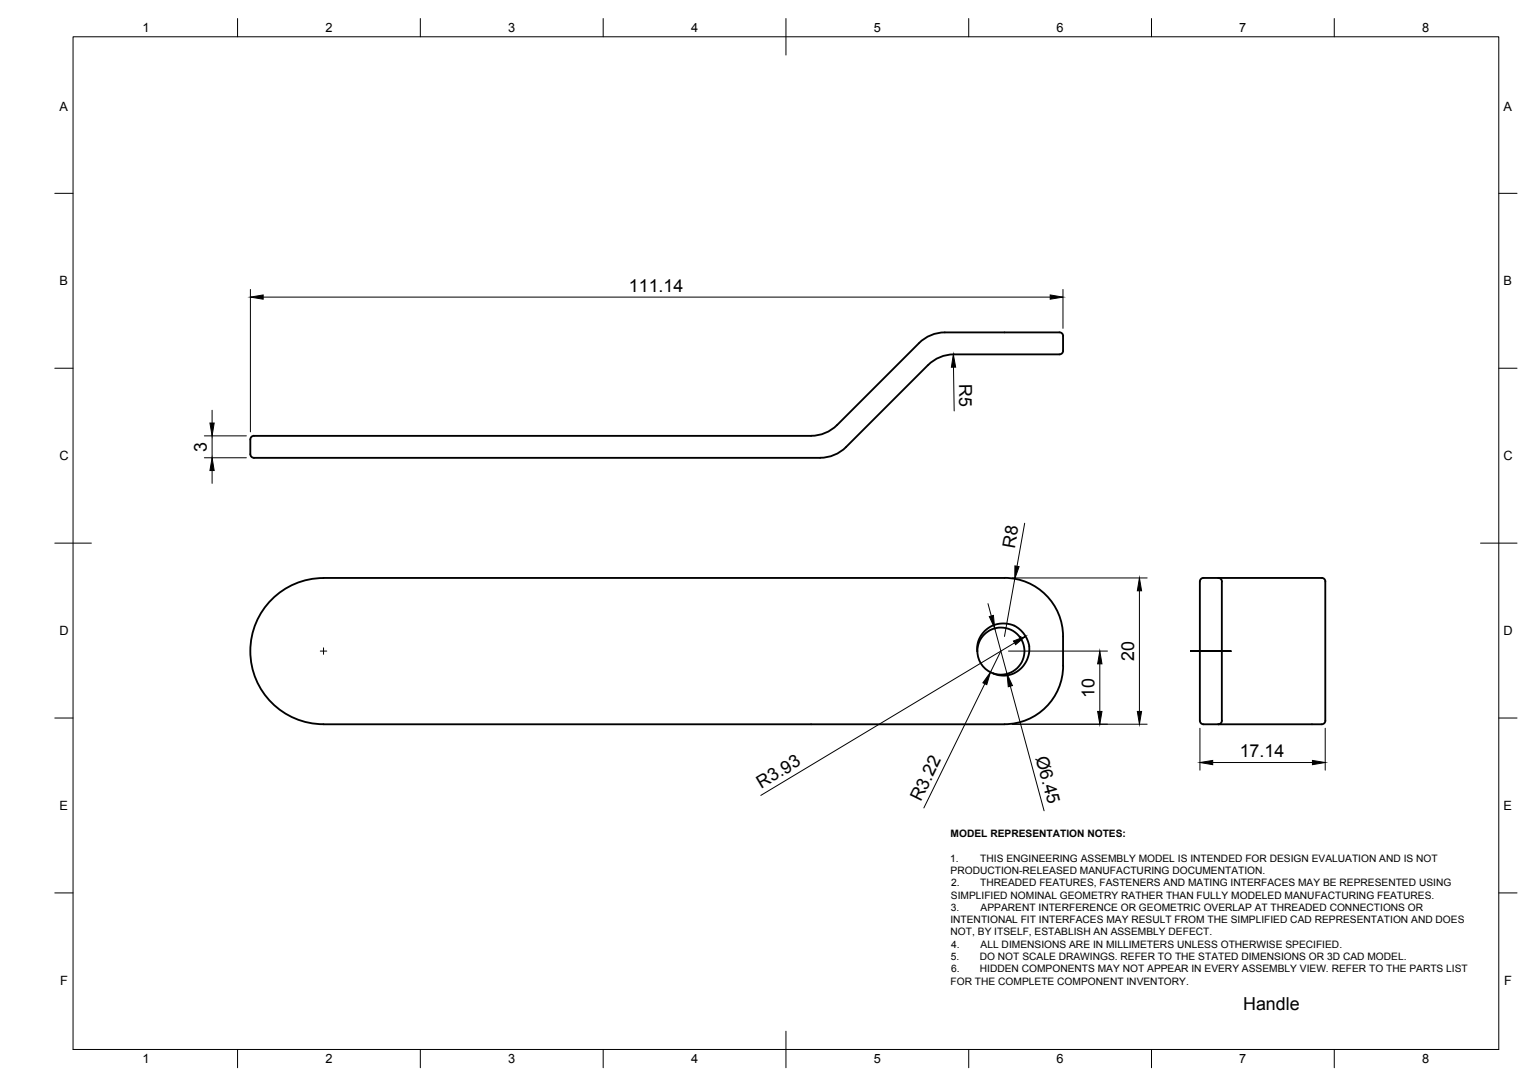
ISO-10303-21;
HEADER;
/* Generated by software containing ST-Developer
 * from STEP Tools, Inc. (www.steptools.com) 
 */

FILE_DESCRIPTION(
/* description */ (''),
/* implementation_level */ '2;1');

FILE_NAME(
/* name */ 'Handle.step',
/* time_stamp */ '2026-10-06T12:47:13-07:00',
/* author */ (''),
/* organization */ (''),
/* preprocessor_version */ 'ST-DEVELOPER v20.2',
/* originating_system */ 'Autodesk Translation Framework v15.15.0.0',
/* authorisation */ '');

FILE_SCHEMA (('AUTOMOTIVE_DESIGN { 1 0 10303 214 3 1 1 }'));
ENDSEC;

DATA;
#10=MECHANICAL_DESIGN_GEOMETRIC_PRESENTATION_REPRESENTATION('',(#74),#42667);
#56=SHAPE_REPRESENTATION_RELATIONSHIP('SRR','None',#42709,#65);
#65=ADVANCED_BREP_SHAPE_REPRESENTATION('',(#83),#42665);
#74=STYLED_ITEM('',(#42756),#83);
#83=MANIFOLD_SOLID_BREP('Body1',#4039);
#90=B_SPLINE_SURFACE_WITH_KNOTS('',3,3,((#34754,#34755,#34756,#34757,#34758,
#34759,#34760,#34761,#34762,#34763,#34764,#34765,#34766,#34767,#34768,#34769,
#34770,#34771,#34772,#34773,#34774,#34775,#34776,#34777,#34778,#34779,#34780,
#34781,#34782,#34783,#34784,#34785,#34786,#34787,#34788,#34789,#34790,#34791,
#34792,#34793,#34794,#34795,#34796,#34797,#34798,#34799,#34800,#34801,#34802,
#34803,#34804,#34805,#34806,#34807,#34808,#34809,#34810,#34811,#34812,#34813,
#34814,#34815,#34816,#34817,#34818,#34819,#34820,#34821,#34822,#34823,#34824,
#34825,#34826,#34827,#34828,#34829,#34830,#34831,#34832,#34833,#34834,#34835,
#34836,#34837,#34838,#34839,#34840,#34841,#34842,#34843,#34844,#34845,#34846,
#34847,#34848,#34849,#34850,#34851,#34852,#34853,#34854,#34855,#34856,#34857,
#34858,#34859,#34860,#34861,#34862,#34863,#34864,#34865,#34866,#34867,#34868,
#34869,#34870,#34871,#34872,#34873,#34874,#34875,#34876,#34877,#34878,#34879,
#34880,#34881,#34882,#34883,#34884,#34885,#34886,#34887,#34888,#34889,#34890,
#34891,#34892,#34893,#34894,#34895,#34896,#34897,#34898,#34899,#34900,#34901,
#34902,#34903,#34904,#34905,#34906,#34907,#34908,#34909,#34910,#34911,#34912,
#34913,#34914,#34915,#34916,#34917,#34918,#34919,#34920,#34921,#34922,#34923,
#34924,#34925,#34926,#34927,#34928,#34929,#34930,#34931,#34932,#34933,#34934),
(#34935,#34936,#34937,#34938,#34939,#34940,#34941,#34942,#34943,#34944,
#34945,#34946,#34947,#34948,#34949,#34950,#34951,#34952,#34953,#34954,#34955,
#34956,#34957,#34958,#34959,#34960,#34961,#34962,#34963,#34964,#34965,#34966,
#34967,#34968,#34969,#34970,#34971,#34972,#34973,#34974,#34975,#34976,#34977,
#34978,#34979,#34980,#34981,#34982,#34983,#34984,#34985,#34986,#34987,#34988,
#34989,#34990,#34991,#34992,#34993,#34994,#34995,#34996,#34997,#34998,#34999,
#35000,#35001,#35002,#35003,#35004,#35005,#35006,#35007,#35008,#35009,#35010,
#35011,#35012,#35013,#35014,#35015,#35016,#35017,#35018,#35019,#35020,#35021,
#35022,#35023,#35024,#35025,#35026,#35027,#35028,#35029,#35030,#35031,#35032,
#35033,#35034,#35035,#35036,#35037,#35038,#35039,#35040,#35041,#35042,#35043,
#35044,#35045,#35046,#35047,#35048,#35049,#35050,#35051,#35052,#35053,#35054,
#35055,#35056,#35057,#35058,#35059,#35060,#35061,#35062,#35063,#35064,#35065,
#35066,#35067,#35068,#35069,#35070,#35071,#35072,#35073,#35074,#35075,#35076,
#35077,#35078,#35079,#35080,#35081,#35082,#35083,#35084,#35085,#35086,#35087,
#35088,#35089,#35090,#35091,#35092,#35093,#35094,#35095,#35096,#35097,#35098,
#35099,#35100,#35101,#35102,#35103,#35104,#35105,#35106,#35107,#35108,#35109,
#35110,#35111,#35112,#35113,#35114,#35115),(#35116,#35117,#35118,#35119,
#35120,#35121,#35122,#35123,#35124,#35125,#35126,#35127,#35128,#35129,#35130,
#35131,#35132,#35133,#35134,#35135,#35136,#35137,#35138,#35139,#35140,#35141,
#35142,#35143,#35144,#35145,#35146,#35147,#35148,#35149,#35150,#35151,#35152,
#35153,#35154,#35155,#35156,#35157,#35158,#35159,#35160,#35161,#35162,#35163,
#35164,#35165,#35166,#35167,#35168,#35169,#35170,#35171,#35172,#35173,#35174,
#35175,#35176,#35177,#35178,#35179,#35180,#35181,#35182,#35183,#35184,#35185,
#35186,#35187,#35188,#35189,#35190,#35191,#35192,#35193,#35194,#35195,#35196,
#35197,#35198,#35199,#35200,#35201,#35202,#35203,#35204,#35205,#35206,#35207,
#35208,#35209,#35210,#35211,#35212,#35213,#35214,#35215,#35216,#35217,#35218,
#35219,#35220,#35221,#35222,#35223,#35224,#35225,#35226,#35227,#35228,#35229,
#35230,#35231,#35232,#35233,#35234,#35235,#35236,#35237,#35238,#35239,#35240,
#35241,#35242,#35243,#35244,#35245,#35246,#35247,#35248,#35249,#35250,#35251,
#35252,#35253,#35254,#35255,#35256,#35257,#35258,#35259,#35260,#35261,#35262,
#35263,#35264,#35265,#35266,#35267,#35268,#35269,#35270,#35271,#35272,#35273,
#35274,#35275,#35276,#35277,#35278,#35279,#35280,#35281,#35282,#35283,#35284,
#35285,#35286,#35287,#35288,#35289,#35290,#35291,#35292,#35293,#35294,#35295,
#35296),(#35297,#35298,#35299,#35300,#35301,#35302,#35303,#35304,#35305,
#35306,#35307,#35308,#35309,#35310,#35311,#35312,#35313,#35314,#35315,#35316,
#35317,#35318,#35319,#35320,#35321,#35322,#35323,#35324,#35325,#35326,#35327,
#35328,#35329,#35330,#35331,#35332,#35333,#35334,#35335,#35336,#35337,#35338,
#35339,#35340,#35341,#35342,#35343,#35344,#35345,#35346,#35347,#35348,#35349,
#35350,#35351,#35352,#35353,#35354,#35355,#35356,#35357,#35358,#35359,#35360,
#35361,#35362,#35363,#35364,#35365,#35366,#35367,#35368,#35369,#35370,#35371,
#35372,#35373,#35374,#35375,#35376,#35377,#35378,#35379,#35380,#35381,#35382,
#35383,#35384,#35385,#35386,#35387,#35388,#35389,#35390,#35391,#35392,#35393,
#35394,#35395,#35396,#35397,#35398,#35399,#35400,#35401,#35402,#35403,#35404,
#35405,#35406,#35407,#35408,#35409,#35410,#35411,#35412,#35413,#35414,#35415,
#35416,#35417,#35418,#35419,#35420,#35421,#35422,#35423,#35424,#35425,#35426,
#35427,#35428,#35429,#35430,#35431,#35432,#35433,#35434,#35435,#35436,#35437,
#35438,#35439,#35440,#35441,#35442,#35443,#35444,#35445,#35446,#35447,#35448,
#35449,#35450,#35451,#35452,#35453,#35454,#35455,#35456,#35457,#35458,#35459,
#35460,#35461,#35462,#35463,#35464,#35465,#35466,#35467,#35468,#35469,#35470,
#35471,#35472,#35473,#35474,#35475,#35476,#35477)),.UNSPECIFIED.,.F.,.F.,
 .F.,(4,4),(4,1,1,1,1,1,1,1,1,1,1,1,1,1,1,1,1,1,1,1,1,1,1,1,1,1,1,1,1,1,
1,1,1,1,1,1,1,1,1,1,1,1,1,1,1,1,1,1,1,1,1,1,1,1,1,1,1,1,1,1,1,1,1,1,1,1,
1,1,1,1,1,1,1,1,1,1,1,1,1,1,1,1,1,1,1,1,1,1,1,1,1,1,1,1,1,1,1,1,1,1,1,1,
1,1,1,1,1,1,1,1,1,1,1,1,1,1,1,1,1,1,1,1,1,1,1,1,1,1,1,1,1,1,1,1,1,1,1,1,
1,1,1,1,1,1,1,1,1,1,1,1,1,1,1,1,1,1,1,1,1,1,1,1,1,1,1,1,1,1,1,1,1,1,1,1,
1,1,1,1,4),(-0.000650925100349628,0.0823958707828885),(8.31473274985812,
9.3146787622095,10.3146247745609,11.3145707869122,12.3145167992636,13.314462811615,
14.3144088239664,15.3143548363177,16.3143008486691,17.3142468610205,18.3141928733718,
19.3141388857232,20.3140848980746,21.314030910426,22.3139769227773,23.3139229351287,
24.3138689474801,25.3138149598315,26.3137609721828,27.3137069845342,28.3136529968856,
29.3135990092369,30.3135450215883,31.3134910339397,32.3134370462911,33.3133830586424,
34.3133290709938,35.3132750833452,36.3132210956965,37.3131671080479,38.3131131203993,
39.3130591327507,40.313005145102,41.3129511574534,42.3128971698048,43.3128431821562,
44.3127891945075,45.3127352068589,46.3126812192103,47.3126272315616,48.312573243913,
49.3125192562644,50.3124652686158,51.3124112809671,52.3123572933185,53.3123033056699,
54.3122493180213,55.3121953303726,56.312141342724,57.3120873550754,58.3120333674267,
59.3119793797781,60.3119253921295,61.3118714044809,62.3118174168322,63.3117634291836,
64.311709441535,65.3116554538863,66.3116014662377,67.3115474785891,68.3114934909405,
69.3114395032918,70.3113855156432,71.3113315279946,72.311277540346,73.3112235526973,
74.3111695650487,75.3111155774001,76.3110615897514,77.3110076021028,78.3109536144542,
79.3108996268056,80.3108456391569,81.3107916515083,82.3107376638597,83.3106836762111,
84.3106296885624,85.3105757009138,86.3105217132652,87.3104677256165,88.3104137379679,
89.3103597503193,90.3103057626707,91.310251775022,92.3101977873734,93.3101437997248,
94.3100898120761,95.3100358244275,96.3099818367789,97.3099278491303,98.3098738614816,
99.309819873833,100.309765886184,101.309711898536,102.309657910887,103.309603923238,
104.30954993559,105.309495947941,106.309441960293,107.309387972644,108.309333984995,
109.309279997347,110.309226009698,111.309172022049,112.309118034401,113.309064046752,
114.309010059104,115.308956071455,116.308902083806,117.308848096158,118.308794108509,
119.30874012086,120.308686133212,121.308632145563,122.308578157915,123.308524170266,
124.308470182617,125.308416194969,126.30836220732,127.308308219671,128.308254232023,
129.308200244374,130.308146256726,131.308092269077,132.308038281428,133.30798429378,
134.307930306131,135.307876318482,136.307822330834,137.307768343185,138.307714355537,
139.307660367888,140.307606380239,141.307552392591,142.307498404942,143.307444417293,
144.307390429645,145.307336441996,146.307282454348,147.307228466699,148.30717447905,
149.307120491402,150.307066503753,151.307012516104,152.306958528456,153.306904540807,
154.306850553158,155.30679656551,156.306742577861,157.306688590213,158.306634602564,
159.306580614915,160.306526627267,161.306472639618,162.306418651969,163.306364664321,
164.306310676672,165.306256689024,166.306202701375,167.306148713726,168.306094726078,
169.306040738429,170.30598675078,171.305932763132,172.305878775483,173.305824787835,
174.305770800186,175.305716812537,176.305662824889,177.30560883724,178.305554849591,
179.305500861943,180.305446874294,181.305392886646,182.305338898997,183.305284911348,
184.3052309237,185.305176936051,186.305773873502),.UNSPECIFIED.);
#91=B_SPLINE_SURFACE_WITH_KNOTS('',3,3,((#35967,#35968,#35969,#35970,#35971,
#35972,#35973,#35974,#35975,#35976,#35977,#35978,#35979,#35980,#35981,#35982,
#35983,#35984,#35985,#35986,#35987,#35988,#35989,#35990,#35991,#35992,#35993,
#35994,#35995,#35996,#35997,#35998,#35999,#36000,#36001,#36002,#36003,#36004,
#36005,#36006,#36007,#36008,#36009,#36010,#36011,#36012,#36013,#36014,#36015,
#36016,#36017,#36018,#36019,#36020,#36021,#36022,#36023,#36024,#36025,#36026,
#36027,#36028,#36029,#36030,#36031,#36032,#36033,#36034,#36035,#36036,#36037,
#36038,#36039,#36040,#36041,#36042,#36043,#36044,#36045,#36046,#36047,#36048,
#36049,#36050,#36051,#36052,#36053,#36054,#36055,#36056,#36057,#36058,#36059,
#36060,#36061,#36062,#36063,#36064,#36065,#36066,#36067,#36068,#36069,#36070,
#36071,#36072,#36073,#36074,#36075,#36076,#36077,#36078,#36079,#36080,#36081,
#36082,#36083,#36084,#36085,#36086,#36087,#36088,#36089,#36090,#36091,#36092,
#36093,#36094,#36095,#36096,#36097,#36098,#36099,#36100,#36101,#36102,#36103,
#36104,#36105,#36106,#36107,#36108,#36109,#36110,#36111,#36112,#36113,#36114,
#36115,#36116,#36117,#36118,#36119,#36120,#36121,#36122,#36123,#36124,#36125,
#36126,#36127,#36128,#36129,#36130,#36131,#36132,#36133,#36134,#36135,#36136,
#36137,#36138,#36139,#36140,#36141,#36142,#36143,#36144,#36145,#36146,#36147),
(#36148,#36149,#36150,#36151,#36152,#36153,#36154,#36155,#36156,#36157,
#36158,#36159,#36160,#36161,#36162,#36163,#36164,#36165,#36166,#36167,#36168,
#36169,#36170,#36171,#36172,#36173,#36174,#36175,#36176,#36177,#36178,#36179,
#36180,#36181,#36182,#36183,#36184,#36185,#36186,#36187,#36188,#36189,#36190,
#36191,#36192,#36193,#36194,#36195,#36196,#36197,#36198,#36199,#36200,#36201,
#36202,#36203,#36204,#36205,#36206,#36207,#36208,#36209,#36210,#36211,#36212,
#36213,#36214,#36215,#36216,#36217,#36218,#36219,#36220,#36221,#36222,#36223,
#36224,#36225,#36226,#36227,#36228,#36229,#36230,#36231,#36232,#36233,#36234,
#36235,#36236,#36237,#36238,#36239,#36240,#36241,#36242,#36243,#36244,#36245,
#36246,#36247,#36248,#36249,#36250,#36251,#36252,#36253,#36254,#36255,#36256,
#36257,#36258,#36259,#36260,#36261,#36262,#36263,#36264,#36265,#36266,#36267,
#36268,#36269,#36270,#36271,#36272,#36273,#36274,#36275,#36276,#36277,#36278,
#36279,#36280,#36281,#36282,#36283,#36284,#36285,#36286,#36287,#36288,#36289,
#36290,#36291,#36292,#36293,#36294,#36295,#36296,#36297,#36298,#36299,#36300,
#36301,#36302,#36303,#36304,#36305,#36306,#36307,#36308,#36309,#36310,#36311,
#36312,#36313,#36314,#36315,#36316,#36317,#36318,#36319,#36320,#36321,#36322,
#36323,#36324,#36325,#36326,#36327,#36328),(#36329,#36330,#36331,#36332,
#36333,#36334,#36335,#36336,#36337,#36338,#36339,#36340,#36341,#36342,#36343,
#36344,#36345,#36346,#36347,#36348,#36349,#36350,#36351,#36352,#36353,#36354,
#36355,#36356,#36357,#36358,#36359,#36360,#36361,#36362,#36363,#36364,#36365,
#36366,#36367,#36368,#36369,#36370,#36371,#36372,#36373,#36374,#36375,#36376,
#36377,#36378,#36379,#36380,#36381,#36382,#36383,#36384,#36385,#36386,#36387,
#36388,#36389,#36390,#36391,#36392,#36393,#36394,#36395,#36396,#36397,#36398,
#36399,#36400,#36401,#36402,#36403,#36404,#36405,#36406,#36407,#36408,#36409,
#36410,#36411,#36412,#36413,#36414,#36415,#36416,#36417,#36418,#36419,#36420,
#36421,#36422,#36423,#36424,#36425,#36426,#36427,#36428,#36429,#36430,#36431,
#36432,#36433,#36434,#36435,#36436,#36437,#36438,#36439,#36440,#36441,#36442,
#36443,#36444,#36445,#36446,#36447,#36448,#36449,#36450,#36451,#36452,#36453,
#36454,#36455,#36456,#36457,#36458,#36459,#36460,#36461,#36462,#36463,#36464,
#36465,#36466,#36467,#36468,#36469,#36470,#36471,#36472,#36473,#36474,#36475,
#36476,#36477,#36478,#36479,#36480,#36481,#36482,#36483,#36484,#36485,#36486,
#36487,#36488,#36489,#36490,#36491,#36492,#36493,#36494,#36495,#36496,#36497,
#36498,#36499,#36500,#36501,#36502,#36503,#36504,#36505,#36506,#36507,#36508,
#36509),(#36510,#36511,#36512,#36513,#36514,#36515,#36516,#36517,#36518,
#36519,#36520,#36521,#36522,#36523,#36524,#36525,#36526,#36527,#36528,#36529,
#36530,#36531,#36532,#36533,#36534,#36535,#36536,#36537,#36538,#36539,#36540,
#36541,#36542,#36543,#36544,#36545,#36546,#36547,#36548,#36549,#36550,#36551,
#36552,#36553,#36554,#36555,#36556,#36557,#36558,#36559,#36560,#36561,#36562,
#36563,#36564,#36565,#36566,#36567,#36568,#36569,#36570,#36571,#36572,#36573,
#36574,#36575,#36576,#36577,#36578,#36579,#36580,#36581,#36582,#36583,#36584,
#36585,#36586,#36587,#36588,#36589,#36590,#36591,#36592,#36593,#36594,#36595,
#36596,#36597,#36598,#36599,#36600,#36601,#36602,#36603,#36604,#36605,#36606,
#36607,#36608,#36609,#36610,#36611,#36612,#36613,#36614,#36615,#36616,#36617,
#36618,#36619,#36620,#36621,#36622,#36623,#36624,#36625,#36626,#36627,#36628,
#36629,#36630,#36631,#36632,#36633,#36634,#36635,#36636,#36637,#36638,#36639,
#36640,#36641,#36642,#36643,#36644,#36645,#36646,#36647,#36648,#36649,#36650,
#36651,#36652,#36653,#36654,#36655,#36656,#36657,#36658,#36659,#36660,#36661,
#36662,#36663,#36664,#36665,#36666,#36667,#36668,#36669,#36670,#36671,#36672,
#36673,#36674,#36675,#36676,#36677,#36678,#36679,#36680,#36681,#36682,#36683,
#36684,#36685,#36686,#36687,#36688,#36689,#36690)),.UNSPECIFIED.,.F.,.F.,
 .F.,(4,4),(4,1,1,1,1,1,1,1,1,1,1,1,1,1,1,1,1,1,1,1,1,1,1,1,1,1,1,1,1,1,
1,1,1,1,1,1,1,1,1,1,1,1,1,1,1,1,1,1,1,1,1,1,1,1,1,1,1,1,1,1,1,1,1,1,1,1,
1,1,1,1,1,1,1,1,1,1,1,1,1,1,1,1,1,1,1,1,1,1,1,1,1,1,1,1,1,1,1,1,1,1,1,1,
1,1,1,1,1,1,1,1,1,1,1,1,1,1,1,1,1,1,1,1,1,1,1,1,1,1,1,1,1,1,1,1,1,1,1,1,
1,1,1,1,1,1,1,1,1,1,1,1,1,1,1,1,1,1,1,1,1,1,1,1,1,1,1,1,1,1,1,1,1,1,1,1,
1,1,1,1,4),(-0.00033399260015787,0.082683618112034),(11.6145432153813,12.6151602401062,
13.6151062524576,14.615052264809,15.6149982771603,16.6149442895117,17.6148903018631,
18.6148363142145,19.6147823265658,20.6147283389172,21.6146743512686,22.61462036362,
23.6145663759713,24.6145123883227,25.6144584006741,26.6144044130254,27.6143504253768,
28.6142964377282,29.6142424500796,30.6141884624309,31.6141344747823,32.6140804871337,
33.614026499485,34.6139725118364,35.6139185241878,36.6138645365392,37.6138105488905,
38.6137565612419,39.6137025735933,40.6136485859447,41.613594598296,42.6135406106474,
43.6134866229988,44.6134326353501,45.6133786477015,46.6133246600529,47.6132706724043,
48.6132166847556,49.613162697107,50.6131087094584,51.6130547218097,52.6130007341611,
53.6129467465125,54.6128927588639,55.6128387712152,56.6127847835666,57.612730795918,
58.6126768082694,59.6126228206207,60.6125688329721,61.6125148453235,62.6124608576748,
63.6124068700262,64.6123528823776,65.612298894729,66.6122449070803,67.6121909194317,
68.6121369317831,69.6120829441344,70.6120289564858,71.6119749688372,72.6119209811886,
73.6118669935399,74.6118130058913,75.6117590182427,76.6117050305941,77.6116510429454,
78.6115970552968,79.6115430676482,80.6114890799995,81.6114350923509,82.6113811047023,
83.6113271170537,84.611273129405,85.6112191417564,86.6111651541078,87.6111111664591,
88.6110571788105,89.6110031911619,90.6109492035133,91.6108952158646,92.610841228216,
93.6107872405674,94.6107332529187,95.6106792652701,96.6106252776215,97.6105712899729,
98.6105173023242,99.6104633146756,100.610409327027,101.610355339378,102.61030135173,
103.610247364081,104.610193376432,105.610139388784,106.610085401135,107.610031413487,
108.609977425838,109.609923438189,110.609869450541,111.609815462892,112.609761475243,
113.609707487595,114.609653499946,115.609599512298,116.609545524649,117.609491537,
118.609437549352,119.609383561703,120.609329574054,121.609275586406,122.609221598757,
123.609167611109,124.60911362346,125.609059635811,126.609005648163,127.608951660514,
128.608897672865,129.608843685217,130.608789697568,131.60873570992,132.608681722271,
133.608627734622,134.608573746974,135.608519759325,136.608465771676,137.608411784028,
138.608357796379,139.60830380873,140.608249821082,141.608195833433,142.608141845785,
143.608087858136,144.608033870487,145.607979882839,146.60792589519,147.607871907541,
148.607817919893,149.607763932244,150.607709944596,151.607655956947,152.607601969298,
153.60754798165,154.607493994001,155.607440006352,156.607386018704,157.607332031055,
158.607278043407,159.607224055758,160.607170068109,161.607116080461,162.607062092812,
163.607008105163,164.606954117515,165.606900129866,166.606846142218,167.606792154569,
168.60673816692,169.606684179272,170.606630191623,171.606576203974,172.606522216326,
173.606468228677,174.606414241029,175.60636025338,176.606306265731,177.606252278083,
178.606198290434,179.606144302785,180.606090315137,181.606036327488,182.605982339839,
183.605928352191,184.605874364542,185.605820376894,186.605766389245,187.605712401596,
188.605658413948,189.605604426299),.UNSPECIFIED.);
#304=B_SPLINE_CURVE_WITH_KNOTS('',3,(#33626,#33627,#33628,#33629,#33630,
#33631,#33632,#33633,#33634,#33635,#33636,#33637,#33638,#33639,#33640,#33641,
#33642,#33643,#33644,#33645,#33646,#33647,#33648,#33649,#33650,#33651,#33652,
#33653,#33654,#33655,#33656,#33657,#33658,#33659,#33660,#33661,#33662,#33663,
#33664,#33665,#33666,#33667,#33668,#33669,#33670,#33671,#33672,#33673,#33674,
#33675,#33676,#33677,#33678,#33679,#33680,#33681,#33682,#33683,#33684,#33685,
#33686,#33687,#33688,#33689,#33690,#33691,#33692,#33693,#33694,#33695,#33696,
#33697,#33698,#33699,#33700,#33701,#33702,#33703,#33704,#33705,#33706,#33707,
#33708,#33709,#33710,#33711,#33712,#33713,#33714,#33715,#33716,#33717,#33718,
#33719,#33720,#33721,#33722,#33723,#33724,#33725,#33726,#33727,#33728,#33729,
#33730,#33731),.UNSPECIFIED.,.F.,.F.,(4,3,3,3,3,3,3,3,3,3,3,3,3,3,3,3,3,
3,3,3,3,3,3,3,3,3,3,3,3,3,3,3,3,3,3,4),(-157.874592628305,-157.786189611785,
-157.697869990434,-157.609576734025,-157.521341336046,-157.433113405113,
-157.344871570897,-157.256534662964,-157.168154411437,-157.079625306774,
-156.991523939165,-156.902974396096,-156.814539659262,-156.726195920889,
-156.634368671629,-156.546127348114,-156.457899483313,-156.369663705481,
-156.281398642303,-156.193033160389,-156.104608179461,-156.016052750418,
-155.991577926814,-155.903028384309,-155.814593648058,-155.726249910282,
-155.634422660805,-155.546181337927,-155.457953473776,-155.369717696606,
-155.281452634103,-155.193087152878,-155.104662172649,-155.016106744312,
-154.991631914463,-154.889196412504),.UNSPECIFIED.);
#305=B_SPLINE_CURVE_WITH_KNOTS('',3,(#33734,#33735,#33736,#33737,#33738,
#33739,#33740,#33741,#33742,#33743,#33744,#33745,#33746,#33747,#33748,#33749,
#33750,#33751,#33752,#33753,#33754,#33755,#33756,#33757,#33758,#33759,#33760,
#33761,#33762,#33763,#33764,#33765,#33766,#33767,#33768,#33769,#33770,#33771,
#33772,#33773,#33774,#33775,#33776,#33777,#33778,#33779,#33780,#33781,#33782,
#33783,#33784,#33785,#33786,#33787,#33788,#33789,#33790,#33791,#33792,#33793,
#33794,#33795,#33796,#33797,#33798,#33799,#33800,#33801,#33802,#33803,#33804,
#33805,#33806,#33807,#33808,#33809,#33810,#33811,#33812,#33813,#33814,#33815,
#33816,#33817,#33818,#33819,#33820,#33821,#33822,#33823,#33824,#33825,#33826,
#33827,#33828,#33829,#33830,#33831,#33832,#33833,#33834,#33835,#33836,#33837,
#33838,#33839,#33840,#33841,#33842,#33843,#33844,#33845,#33846,#33847,#33848,
#33849,#33850,#33851,#33852,#33853,#33854,#33855,#33856,#33857,#33858,#33859,
#33860,#33861,#33862,#33863,#33864,#33865,#33866,#33867,#33868,#33869,#33870,
#33871,#33872,#33873,#33874,#33875),.UNSPECIFIED.,.F.,.F.,(4,3,3,3,3,3,
3,3,3,3,3,3,3,3,3,3,3,3,3,3,3,3,3,3,3,3,3,3,3,3,3,3,3,3,3,3,3,3,3,3,3,3,
3,3,3,3,3,4),(151.906492583222,151.991793877409,152.080343420566,152.168778157483,
152.257121895935,152.348949145163,152.437190468744,152.525418333606,152.613654111494,
152.701919174722,152.790284656678,152.878709637644,152.967265066718,152.99173988976,
153.080289432964,153.168724169926,153.257067908422,153.348895157633,153.437136481254,
153.525364346154,153.61360012408,153.701865187344,153.790230669334,153.878655650331,
153.967211079435,153.991685902111,154.08023544587,154.16867018339,154.257013922446,
154.348841171448,154.43708249563,154.52531036109,154.613546139575,154.701811203397,
154.790176685939,154.878601667486,154.967157097132,154.991631914463,155.080192114906,
155.173042552799,155.261373796928,155.349645458985,155.437878960375,155.526095688543,
155.614346382667,155.702616937377,155.790964593394,155.822995618054),
 .UNSPECIFIED.);
#306=B_SPLINE_CURVE_WITH_KNOTS('',3,(#33881,#33882,#33883,#33884,#33885,
#33886,#33887,#33888,#33889,#33890,#33891,#33892,#33893,#33894,#33895,#33896,
#33897,#33898,#33899,#33900,#33901,#33902,#33903,#33904,#33905,#33906,#33907,
#33908,#33909,#33910,#33911,#33912,#33913,#33914,#33915,#33916,#33917,#33918,
#33919,#33920,#33921,#33922,#33923,#33924,#33925,#33926,#33927,#33928,#33929,
#33930,#33931,#33932,#33933,#33934,#33935,#33936,#33937,#33938,#33939,#33940,
#33941,#33942,#33943,#33944,#33945,#33946,#33947,#33948,#33949,#33950,#33951,
#33952,#33953,#33954,#33955,#33956,#33957,#33958,#33959,#33960,#33961,#33962,
#33963,#33964,#33965,#33966,#33967,#33968,#33969,#33970,#33971,#33972,#33973,
#33974,#33975,#33976,#33977,#33978,#33979,#33980,#33981,#33982,#33983,#33984,
#33985,#33986,#33987,#33988,#33989,#33990,#33991,#33992,#33993,#33994,#33995,
#33996,#33997,#33998,#33999,#34000,#34001,#34002,#34003,#34004,#34005,#34006,
#34007,#34008,#34009,#34010,#34011,#34012,#34013,#34014,#34015,#34016,#34017,
#34018,#34019,#34020,#34021,#34022,#34023,#34024,#34025,#34026,#34027,#34028,
#34029,#34030,#34031,#34032,#34033,#34034,#34035,#34036,#34037,#34038,#34039,
#34040,#34041,#34042,#34043,#34044,#34045,#34046,#34047,#34048,#34049,#34050,
#34051,#34052,#34053,#34054,#34055),.UNSPECIFIED.,.F.,.F.,(4,3,3,3,3,3,
3,3,3,3,3,3,3,3,3,3,3,3,3,3,3,3,3,3,3,3,3,3,3,3,3,3,3,3,3,3,3,3,3,3,3,3,
3,3,3,3,3,3,3,3,3,3,3,3,3,3,3,3,4),(140.743350880823,140.831741437458,140.920276004824,
140.992387741544,141.080937284805,141.169372021824,141.257715760379,141.349543009569,
141.437784333251,141.526012198212,141.6142479762,141.702513039528,141.790878521581,
141.879303502642,141.96785893181,141.992333753895,142.080883297156,142.169318034175,
142.257661772731,142.34948902192,142.437730345602,142.525958210564,142.614193988552,
142.702459051879,142.790824533932,142.879249514994,142.967804944162,142.992279766246,
143.080829309507,143.169264046527,143.257607785082,143.349435034271,143.437676357953,
143.525904222915,143.614140000903,143.70240506423,143.790770546284,143.879195527345,
143.967750956513,143.992225778598,144.080775321858,144.169210058877,144.257553797432,
144.349381046622,144.437622370303,144.525850235265,144.614086013251,144.702351076578,
144.79071655863,144.879141539691,144.967696968859,144.992171790949,145.081319122906,
145.170348342848,145.259280195558,145.350286965679,145.439082830911,145.531195053476,
145.623307276042),.UNSPECIFIED.);
#307=B_SPLINE_CURVE_WITH_KNOTS('',3,(#34058,#34059,#34060,#34061,#34062,
#34063,#34064,#34065,#34066,#34067,#34068,#34069,#34070,#34071,#34072,#34073,
#34074,#34075,#34076,#34077,#34078,#34079,#34080,#34081,#34082,#34083,#34084,
#34085,#34086,#34087,#34088,#34089,#34090,#34091,#34092,#34093,#34094,#34095,
#34096,#34097,#34098,#34099,#34100,#34101,#34102,#34103,#34104,#34105,#34106,
#34107,#34108,#34109,#34110,#34111,#34112,#34113,#34114,#34115,#34116,#34117,
#34118,#34119,#34120,#34121,#34122,#34123,#34124,#34125,#34126,#34127,#34128,
#34129,#34130,#34131,#34132,#34133,#34134,#34135,#34136,#34137,#34138,#34139,
#34140,#34141,#34142,#34143,#34144,#34145,#34146,#34147,#34148,#34149,#34150,
#34151,#34152,#34153,#34154,#34155,#34156,#34157,#34158,#34159,#34160,#34161,
#34162,#34163,#34164,#34165,#34166,#34167,#34168,#34169,#34170,#34171,#34172,
#34173,#34174,#34175,#34176,#34177,#34178,#34179,#34180,#34181,#34182,#34183,
#34184,#34185,#34186,#34187,#34188,#34189,#34190,#34191,#34192,#34193,#34194,
#34195,#34196,#34197,#34198,#34199,#34200,#34201,#34202,#34203,#34204,#34205,
#34206,#34207,#34208,#34209,#34210,#34211,#34212,#34213,#34214,#34215,#34216,
#34217,#34218,#34219,#34220,#34221,#34222,#34223,#34224,#34225,#34226,#34227,
#34228,#34229,#34230,#34231,#34232,#34233,#34234,#34235,#34236,#34237,#34238,
#34239,#34240,#34241,#34242,#34243,#34244,#34245,#34246,#34247,#34248,#34249,
#34250,#34251,#34252,#34253,#34254,#34255,#34256,#34257,#34258,#34259,#34260,
#34261,#34262,#34263,#34264,#34265,#34266,#34267,#34268),.UNSPECIFIED.,
 .F.,.F.,(4,3,3,3,3,3,3,3,3,3,3,3,3,3,3,3,3,3,3,3,3,3,3,3,3,3,3,3,3,3,3,
3,3,3,3,3,3,3,3,3,3,3,3,3,3,3,3,3,3,3,3,3,3,3,3,3,3,3,3,3,3,3,3,3,3,3,3,
3,3,3,4),(-148.606011105325,-148.516896311246,-148.427765779446,-148.338599573289,
-148.249313397802,-148.159965224952,-148.070452324036,-147.992009828003,
-147.903460284745,-147.815025547728,-147.726681809176,-147.634854559986,
-147.546613236307,-147.458385371348,-147.370149593363,-147.281884530039,
-147.193519047988,-147.10509406693,-147.016538637765,-146.992063815652,
-146.903514272392,-146.815079535374,-146.72673579682,-146.63490854763,-146.546667223949,
-146.458439358988,-146.370203581002,-146.281938517676,-146.193573035624,
-146.105148054564,-146.016592625397,-145.9921178033,-145.903568260038,-145.815133523017,
-145.72678978446,-145.634962535271,-145.546721211588,-145.458493346624,
-145.370257568635,-145.281992505305,-145.19362702325,-145.105202042187,
-145.016646613017,-144.992171790949,-144.903622247689,-144.81518751067,
-144.726843772116,-144.635016522926,-144.546775199245,-144.458547334283,
-144.370311556296,-144.28204649297,-144.193681010918,-144.105256029857,
-144.016700600689,-143.992225778598,-143.903676235337,-143.815241498317,
-143.726897759762,-143.635070510573,-143.54682918689,-143.458601321928,
-143.37036554394,-143.282100480614,-143.193734998561,-143.1053100175,-143.016754588331,
-142.992279766246,-142.903798486074,-142.815448035224,-142.804552478338),
 .UNSPECIFIED.);
#308=B_SPLINE_CURVE_WITH_KNOTS('',3,(#34274,#34275,#34276,#34277,#34278),
 .UNSPECIFIED.,.F.,.F.,(4,1,4),(164.458927397274,165.306256689024,166.198929965428),
 .UNSPECIFIED.);
#309=B_SPLINE_CURVE_WITH_KNOTS('',3,(#34282,#34283,#34284,#34285,#34286,
#34287,#34288,#34289,#34290,#34291,#34292,#34293,#34294,#34295,#34296,#34297,
#34298,#34299,#34300,#34301,#34302,#34303,#34304,#34305,#34306,#34307,#34308,
#34309,#34310,#34311,#34312,#34313,#34314,#34315,#34316,#34317,#34318,#34319,
#34320,#34321),.UNSPECIFIED.,.F.,.F.,(4,2,2,2,2,2,2,2,2,2,2,2,2,2,2,2,2,
2,2,4),(-4.06137411129811,-4.03546814208168,-4.03260936723115,-4.03068543622094,
-4.02910207865154,-4.02742394594966,-4.02528765473165,-4.02188101107949,
-4.00378125912536,-3.99087511127817,-3.92336215122477,-3.89390000861074,
-3.87625324670922,-3.87100804923103,-3.86772941140725,-3.86470704756532,
-3.86081439142151,-3.85437488405435,-3.81121148531092,-3.76149375020669),
 .UNSPECIFIED.);
#310=B_SPLINE_CURVE_WITH_KNOTS('',3,(#34322,#34323,#34324,#34325,#34326,
#34327,#34328,#34329,#34330,#34331,#34332,#34333,#34334,#34335,#34336,#34337,
#34338,#34339,#34340,#34341,#34342,#34343,#34344,#34345,#34346,#34347,#34348,
#34349,#34350,#34351,#34352,#34353,#34354,#34355,#34356,#34357,#34358,#34359,
#34360,#34361,#34362,#34363,#34364,#34365,#34366,#34367,#34368,#34369,#34370,
#34371,#34372,#34373,#34374,#34375,#34376,#34377,#34378,#34379,#34380,#34381,
#34382,#34383,#34384,#34385,#34386,#34387,#34388,#34389,#34390,#34391,#34392,
#34393,#34394,#34395,#34396,#34397,#34398,#34399,#34400,#34401,#34402,#34403,
#34404,#34405,#34406,#34407,#34408,#34409),.UNSPECIFIED.,.F.,.F.,(4,2,2,
2,2,2,2,2,2,2,2,2,2,2,2,2,2,2,2,2,2,2,2,2,2,2,2,2,2,2,2,2,2,2,2,2,2,2,2,
2,2,2,2,4),(-0.662156536932336,-0.648956013746852,-0.621418192193571,-0.617234499775957,
-0.615108581233505,-0.613431055280487,-0.611475622140756,-0.607966632969675,
-0.591020215921372,-0.514722936640716,-0.465485531341795,-0.458903121030178,
-0.454968378544555,-0.451939320614257,-0.448679115744897,-0.443518536519126,
-0.426662623721119,-0.399038694208074,-0.355194168524487,-0.298655849376382,
-0.294253481146245,-0.292112018854427,-0.290433286732513,-0.290426632483179,
-0.290420084506535,-0.290413640687297,-0.290407299018121,-0.290401057478961,
-0.2903949140909,-0.288474887817562,-0.285144057785002,-0.280975459144695,
-0.272195312542459,-0.246600417983609,-0.184345430883523,-0.142200987206802,
-0.135789521101596,-0.13190488755513,-0.128883447241603,-0.125600486147694,
-0.120336747935594,-0.102516454894325,-0.0726393233951299,-0.000963379534404715),
 .UNSPECIFIED.);
#311=B_SPLINE_CURVE_WITH_KNOTS('',3,(#34415,#34416,#34417,#34418,#34419,
#34420,#34421,#34422,#34423,#34424,#34425,#34426,#34427,#34428,#34429,#34430,
#34431,#34432,#34433,#34434,#34435,#34436,#34437,#34438,#34439,#34440,#34441,
#34442,#34443,#34444,#34445,#34446,#34447,#34448,#34449,#34450,#34451,#34452,
#34453,#34454,#34455,#34456,#34457,#34458,#34459,#34460,#34461,#34462,#34463,
#34464,#34465,#34466,#34467,#34468,#34469,#34470,#34471,#34472,#34473,#34474,
#34475,#34476,#34477,#34478,#34479,#34480,#34481,#34482,#34483,#34484,#34485,
#34486,#34487,#34488,#34489,#34490),.UNSPECIFIED.,.F.,.F.,(4,2,2,2,2,2,
2,2,2,2,2,2,2,2,2,2,2,2,2,2,2,2,2,2,2,2,2,2,2,2,2,2,2,2,2,2,2,4),(-4.0614630673581,
-4.05235423870892,-3.96283840444798,-3.93777252469754,-3.93188013811726,
-3.92845778818342,-3.92546300471007,-3.92175396700727,-3.91606035920602,
-3.88902746696132,-3.8050304357142,-3.78310043186638,-3.77517962828362,
-3.77130702260846,-3.76816909778494,-3.76629336885218,-3.76469327318415,
-3.76255009404327,-3.75814060112062,-3.7020680575884,-3.65787276096341,
-3.6302390214585,-3.6133762570027,-3.60821407922187,-3.60495294503442,-3.60192307173183,
-3.59798732806223,-3.59140329432733,-3.54215389317604,-3.4657303365375,
-3.44886309154659,-3.44535811526621,-3.44340319417903,-3.44172502335401,
-3.43959686996878,-3.43540447334862,-3.40763336833459,-3.40023537643569),
 .UNSPECIFIED.);
#312=B_SPLINE_CURVE_WITH_KNOTS('',3,(#34491,#34492,#34493,#34494,#34495,
#34496,#34497,#34498,#34499),.UNSPECIFIED.,.F.,.F.,(4,1,1,1,1,1,4),(160.22122533308,
160.306526627267,161.306472639618,162.306418651969,163.306364664321,164.306310676672,
164.458927397274),.UNSPECIFIED.);
#313=B_SPLINE_CURVE_WITH_KNOTS('',3,(#34500,#34501,#34502,#34503,#34504,
#34505,#34506,#34507,#34508,#34509,#34510,#34511,#34512,#34513,#34514,#34515,
#34516,#34517,#34518,#34519,#34520,#34521,#34522,#34523,#34524,#34525,#34526,
#34527,#34528,#34529,#34530,#34531,#34532,#34533,#34534,#34535,#34536,#34537,
#34538,#34539,#34540,#34541,#34542,#34543,#34544,#34545,#34546,#34547,#34548,
#34549,#34550,#34551,#34552,#34553,#34554,#34555,#34556,#34557,#34558,#34559,
#34560,#34561,#34562,#34563,#34564,#34565,#34566,#34567,#34568,#34569,#34570,
#34571,#34572,#34573,#34574,#34575,#34576,#34577,#34578,#34579,#34580,#34581,
#34582,#34583,#34584,#34585,#34586,#34587,#34588,#34589,#34590,#34591,#34592,
#34593,#34594,#34595,#34596,#34597,#34598,#34599,#34600,#34601,#34602,#34603,
#34604,#34605,#34606,#34607,#34608,#34609,#34610,#34611,#34612,#34613,#34614,
#34615,#34616,#34617,#34618,#34619,#34620,#34621,#34622,#34623,#34624,#34625,
#34626,#34627,#34628,#34629,#34630,#34631,#34632,#34633,#34634,#34635,#34636,
#34637,#34638,#34639,#34640,#34641,#34642,#34643,#34644,#34645,#34646,#34647,
#34648,#34649,#34650,#34651,#34652,#34653,#34654,#34655,#34656,#34657,#34658,
#34659,#34660,#34661,#34662,#34663,#34664,#34665,#34666,#34667,#34668,#34669,
#34670,#34671,#34672,#34673,#34674,#34675,#34676,#34677,#34678,#34679,#34680,
#34681,#34682,#34683,#34684,#34685,#34686,#34687,#34688,#34689,#34690,#34691,
#34692,#34693,#34694,#34695,#34696,#34697,#34698,#34699,#34700,#34701,#34702,
#34703,#34704,#34705,#34706,#34707,#34708,#34709,#34710,#34711),
 .UNSPECIFIED.,.F.,.F.,(4,2,2,2,2,2,2,2,2,2,2,2,2,2,2,2,2,2,2,2,2,2,2,2,
2,2,2,2,2,2,2,2,2,2,2,2,2,2,2,2,2,2,2,2,2,2,2,2,2,2,2,2,2,2,2,2,2,2,2,2,
2,2,2,2,2,2,2,2,2,2,2,2,2,2,2,2,2,2,2,2,2,2,2,2,2,2,2,2,2,2,2,2,2,2,2,2,
2,2,2,2,2,2,2,2,2,4),(-2.69232820337898,-2.65215331755146,-2.57610388787892,
-2.55874252190226,-2.55520845908299,-2.55324739746129,-2.55157016471346,
-2.54945118635699,-2.5453008033091,-2.51868116942949,-2.44436574494018,
-2.41690138391812,-2.40011266218735,-2.39495896467106,-2.391699930452,-2.38866976400286,
-2.38473045818825,-2.37813347333805,-2.32868997370835,-2.25191573891669,
-2.23552390746872,-2.23204851955261,-2.23010018678417,-2.22842149070606,
-2.22628472487605,-2.22287778578281,-2.20478565495202,-2.1045602781164,
-2.07843784358157,-2.07247131749459,-2.06903277073797,-2.06603972630721,
-2.06235328025359,-2.05673239951629,-2.03080471296937,-1.97580982653872,
-1.94588728187544,-1.93779308354745,-1.9134451694628,-1.90938428253259,
-1.90728467757254,-1.90560885148976,-1.90363318936277,-1.90003129527163,
-1.88145719932781,-1.80063827631087,-1.7574399740288,-1.75099908058603,
-1.74710571190354,-1.7440828863301,-1.74080384074389,-1.73555819605331,
-1.71791208240507,-1.68844885628179,-1.63096870377777,-1.59100057425755,
-1.58650919985396,-1.58435018577139,-1.5826697993837,-1.5807373452675,-1.57733328749,
-1.56202461388756,-1.48445088468712,-1.43468019637624,-1.42808727138658,
-1.42414948173725,-1.42111996890225,-1.41786113492771,-1.41270668666146,
-1.39590617689815,-1.36840897502444,-1.29423806712174,-1.26748633929008,
-1.26333151633647,-1.2612117690953,-1.25953470699639,-1.25757473367821,
-1.25404488214976,-1.23674817735237,-1.16070716478711,-1.11159742061136,
-1.10501758302102,-1.10108359618052,-1.09805466260356,-1.0947941410465,
-1.08963210011751,-1.07276280810492,-1.04510818063073,-0.972368929468456,
-0.944493035068862,-0.940299499291466,-0.938171484898872,-0.936493800339113,
-0.934539899570493,-0.931037926828355,-0.914207256388892,-0.837824288323109,
-0.788545872915298,-0.781962655556508,-0.778027682083294,-0.774998593294991,
-0.771738499937146,-0.766578405634705,-0.749726837719345,-0.7221128406229,
-0.662156536932336),.UNSPECIFIED.);
#314=B_SPLINE_CURVE_WITH_KNOTS('',3,(#34718,#34719,#34720,#34721,#34722,
#34723,#34724,#34725,#34726,#34727,#34728,#34729,#34730,#34731,#34732,#34733,
#34734,#34735,#34736,#34737,#34738,#34739,#34740,#34741,#34742,#34743,#34744,
#34745,#34746,#34747,#34748,#34749,#34750,#34751,#34752,#34753),
 .UNSPECIFIED.,.F.,.F.,(4,2,2,2,2,2,2,2,2,2,2,2,2,2,2,2,2,4),(-1.37015241264804,
-1.35570167221927,-1.34911020280277,-1.34517184391813,-1.34214104368373,
-1.33887998266,-1.33372020388906,-1.31688586729512,-1.28931555875076,-1.21574475579553,
-1.18851814157379,-1.18434507533776,-1.18222082213135,-1.18054267426951,
-1.17858425479071,-1.17506423658523,-1.15795382549888,-1.12238864779317),
 .UNSPECIFIED.);
#315=B_SPLINE_CURVE_WITH_KNOTS('',3,(#35478,#35479,#35480,#35481,#35482,
#35483,#35484,#35485,#35486,#35487,#35488,#35489,#35490,#35491),
 .UNSPECIFIED.,.F.,.F.,(4,2,2,2,2,2,4),(0.0079371660209936,0.157935777681907,
0.317600902596195,0.481956426355492,0.644216700819685,0.777027678467974,
0.901017531905197),.UNSPECIFIED.);
#316=B_SPLINE_CURVE_WITH_KNOTS('',3,(#35492,#35493,#35494,#35495,#35496,
#35497,#35498,#35499,#35500,#35501),.UNSPECIFIED.,.F.,.F.,(4,1,1,1,1,1,
1,4),(145.623314962503,145.9921178033,146.992063815652,147.992009828003,
148.991955840354,149.991901852706,150.991847865057,151.906483871255),
 .UNSPECIFIED.);
#317=B_SPLINE_CURVE_WITH_KNOTS('',3,(#35502,#35503,#35504,#35505,#35506,
#35507,#35508,#35509,#35510,#35511,#35512,#35513,#35514,#35515),
 .UNSPECIFIED.,.F.,.F.,(4,2,2,2,2,2,4),(0.0050079574061546,0.120802454330559,
0.259394492895916,0.351675444238468,0.427932493074399,0.483828923769819,
0.523620932636945),.UNSPECIFIED.);
#318=B_SPLINE_CURVE_WITH_KNOTS('',3,(#35516,#35517,#35518,#35519,#35520,
#35521,#35522,#35523,#35524,#35525,#35526,#35527,#35528,#35529,#35530,#35531,
#35532,#35533,#35534,#35535,#35536,#35537,#35538,#35539,#35540,#35541,#35542,
#35543,#35544,#35545,#35546,#35547,#35548,#35549,#35550,#35551,#35552,#35553,
#35554,#35555,#35556,#35557,#35558,#35559,#35560,#35561,#35562,#35563,#35564,
#35565,#35566,#35567,#35568,#35569,#35570,#35571,#35572,#35573,#35574,#35575,
#35576,#35577,#35578,#35579,#35580,#35581,#35582,#35583,#35584,#35585,#35586,
#35587,#35588,#35589,#35590,#35591,#35592,#35593,#35594,#35595,#35596,#35597,
#35598,#35599,#35600,#35601,#35602,#35603,#35604,#35605,#35606,#35607,#35608,
#35609,#35610,#35611,#35612,#35613,#35614,#35615,#35616,#35617,#35618,#35619,
#35620,#35621,#35622,#35623,#35624,#35625,#35626,#35627,#35628,#35629,#35630,
#35631,#35632,#35633,#35634,#35635,#35636,#35637,#35638,#35639,#35640,#35641,
#35642,#35643,#35644,#35645,#35646,#35647,#35648,#35649,#35650,#35651,#35652,
#35653,#35654,#35655,#35656,#35657,#35658,#35659,#35660,#35661,#35662,#35663,
#35664,#35665,#35666,#35667,#35668,#35669,#35670,#35671,#35672,#35673,#35674,
#35675,#35676,#35677,#35678,#35679,#35680,#35681,#35682,#35683,#35684,#35685,
#35686,#35687,#35688,#35689,#35690,#35691,#35692,#35693,#35694,#35695,#35696,
#35697,#35698,#35699,#35700,#35701,#35702,#35703,#35704,#35705,#35706,#35707,
#35708,#35709,#35710,#35711,#35712,#35713,#35714,#35715,#35716,#35717,#35718,
#35719,#35720,#35721,#35722,#35723,#35724,#35725,#35726,#35727,#35728,#35729),
 .UNSPECIFIED.,.F.,.F.,(4,2,2,2,2,2,2,2,2,2,2,2,2,2,2,2,2,2,2,2,2,2,2,2,
2,2,2,2,2,2,2,2,2,2,2,2,2,2,2,2,2,2,2,2,2,2,2,2,2,2,2,2,2,2,2,2,2,2,2,2,
2,2,2,2,2,2,2,2,2,2,2,2,2,2,2,2,2,2,2,2,2,2,2,2,2,2,2,2,2,2,2,2,2,2,2,2,
2,2,2,2,2,2,2,2,2,2,4),(-3.40023537643569,-3.33482078185619,-3.30719486950161,
-3.29033523387914,-3.28517320247625,-3.28191197376044,-3.27888188358579,
-3.27494567499668,-3.26836045983183,-3.21906860335362,-3.1425569306785,
-3.12580076494813,-3.12230240871166,-3.12034886027345,-3.11867042783018,
-3.11654008924492,-3.1123377816331,-3.08421993346944,-3.01182460862819,
-2.98415801707282,-2.96728033953895,-2.96211612285055,-2.95885428238125,
-2.95582415422582,-2.95188864913119,-2.94530626920494,-2.89617337285961,
-2.81998983409003,-2.80278126440513,-2.79925552182887,-2.79729593292003,
-2.79561801718591,-2.7934956514125,-2.78933106242006,-2.76233708521128,
-2.68852255018912,-2.66100033844717,-2.64418544131733,-2.63902794809165,
-2.63576747103202,-2.63273661807035,-2.62879734251646,-2.62220241790063,
-2.57245296636962,-2.49483755632898,-2.47947731681429,-2.47606857340942,
-2.47413450500865,-2.47245336709749,-2.47029422017985,-2.46580539845458,
-2.4262386953559,-2.36847625742542,-2.33896598030259,-2.32129602970495,
-2.31604619892625,-2.3127651407173,-2.30974086132929,-2.30584617027375,
-2.29940420549618,-2.25626330165687,-2.19386345910526,-2.16905381699869,
-2.1561088099532,-2.15288002433365,-2.1509856900146,-2.14929700013531,-2.14710888804055,
-2.14345323594964,-2.12034146941491,-2.10962599753095,-2.03152314379028,
-2.02122744771306,-1.99944375006007,-1.99361917422242,-1.99017733836269,
-1.98718316977388,-1.9834975552179,-1.97637918050148,-1.9200651726639,-1.85963851291728,
-1.83458282172232,-1.83049138590502,-1.82838461643966,-1.8267076302322,
-1.82473587112967,-1.82115458829943,-1.80297942502917,-1.72618180678269,
-1.67871268495384,-1.67216469347124,-1.66823897361453,-1.66521007514229,
-1.66194332995739,-1.65675802400204,-1.6396911344249,-1.6115862890577,-1.54671124652989,
-1.51195632735406,-1.50752256950061,-1.50537423955513,-1.50369411251794,
-1.50175277797187,-1.49831093281251,-1.48245266118319,-1.40528043645708,
-1.37015241264804),.UNSPECIFIED.);
#319=B_SPLINE_CURVE_WITH_KNOTS('',3,(#35732,#35733,#35734,#35735,#35736,
#35737,#35738,#35739,#35740,#35741,#35742,#35743,#35744,#35745,#35746,#35747,
#35748,#35749,#35750,#35751,#35752,#35753,#35754,#35755,#35756,#35757,#35758,
#35759,#35760,#35761,#35762,#35763,#35764,#35765,#35766,#35767,#35768,#35769,
#35770,#35771,#35772,#35773,#35774,#35775,#35776,#35777,#35778,#35779,#35780,
#35781,#35782,#35783,#35784,#35785,#35786,#35787,#35788,#35789,#35790,#35791,
#35792,#35793,#35794,#35795,#35796,#35797,#35798,#35799,#35800,#35801,#35802,
#35803,#35804,#35805,#35806,#35807,#35808,#35809,#35810,#35811,#35812,#35813,
#35814,#35815,#35816,#35817,#35818,#35819,#35820,#35821,#35822,#35823,#35824,
#35825,#35826,#35827,#35828,#35829,#35830,#35831,#35832,#35833,#35834,#35835,
#35836,#35837,#35838,#35839,#35840,#35841,#35842,#35843,#35844,#35845,#35846,
#35847,#35848,#35849,#35850,#35851,#35852,#35853,#35854,#35855,#35856,#35857,
#35858,#35859,#35860,#35861,#35862,#35863,#35864,#35865,#35866,#35867,#35868,
#35869,#35870,#35871,#35872,#35873,#35874,#35875,#35876,#35877,#35878,#35879,
#35880,#35881,#35882,#35883,#35884,#35885,#35886,#35887,#35888,#35889,#35890,
#35891,#35892,#35893,#35894,#35895),.UNSPECIFIED.,.F.,.F.,(4,2,2,2,2,2,
2,2,2,2,2,2,2,2,2,2,2,2,2,2,2,2,2,2,2,2,2,2,2,2,2,2,2,2,2,2,2,2,2,2,2,2,
2,2,2,2,2,2,2,2,2,2,2,2,2,2,2,2,2,2,2,2,2,2,2,2,2,2,2,2,2,2,2,2,2,2,2,2,
2,2,2,4),(-4.0614287578822,-4.03248871540076,-4.01846104360662,-4.01365489798641,
-4.01033316269565,-4.00752181880818,-4.00452327004274,-4.0007622030692,
-3.99489804196461,-3.96524899606189,-3.94584283611108,-3.88111634163756,
-3.85452293802728,-3.84879489543677,-3.84641168900244,-3.84469933804932,
-3.84309929440734,-3.84039647146944,-3.8331451375629,-3.77212380131558,
-3.72144008924457,-3.70353835756497,-3.69530252279819,-3.68872717556511,
-3.68517352177786,-3.68247422333838,-3.67909297441338,-3.67338468946435,
-3.65345836652772,-3.55643899838608,-3.53774678690756,-3.53064256320669,
-3.52546566485076,-3.52317800715839,-3.52148127783768,-3.5196194663786,
-3.51653417352629,-3.50641678134479,-3.50451420221678,-3.41361908352743,
-3.38615026898234,-3.36936041640254,-3.36420716022018,-3.36094858742808,
-3.35791897603315,-3.35398057099992,-3.34738549014509,-3.29815696099868,
-3.22183041738727,-3.20486364478017,-3.2013533191308,-3.1993975661187,-3.19772002182691,
-3.19559442110385,-3.19141237522778,-3.16388011103469,-3.09076122624934,
-3.06315893043958,-3.04631045962763,-3.04115055523152,-3.03789039483268,
-3.03486111368623,-3.03092570368943,-3.02434129471597,-2.97503329712059,
-2.89858817553595,-2.8817742661767,-2.87827305475125,-2.87631921920786,
-2.87464136090194,-2.87251284295468,-2.86831745264589,-2.84038932807227,
-2.76775598971946,-2.74010440623786,-2.72323413696449,-2.71807163743497,
-2.71481077727113,-2.71178149438938,-2.70784700259689,-2.70126615755269,
-2.69232820337898),.UNSPECIFIED.);
#320=B_SPLINE_CURVE_WITH_KNOTS('',3,(#35897,#35898,#35899,#35900,#35901,
#35902,#35903,#35904,#35905,#35906,#35907,#35908,#35909,#35910,#35911,#35912,
#35913,#35914,#35915,#35916,#35917,#35918,#35919,#35920,#35921,#35922,#35923,
#35924,#35925,#35926,#35927,#35928,#35929,#35930,#35931,#35932,#35933,#35934,
#35935,#35936,#35937,#35938,#35939,#35940,#35941,#35942,#35943,#35944,#35945,
#35946,#35947,#35948,#35949,#35950,#35951,#35952,#35953,#35954),
 .UNSPECIFIED.,.F.,.F.,(4,2,2,2,2,2,2,2,2,2,2,2,2,2,2,2,2,2,2,2,2,2,2,2,
2,2,2,2,4),(-0.510303440387924,-0.468140561817124,-0.462130454299904,-0.437689929728706,
-0.433625192760907,-0.431524767779201,-0.429848909425109,-0.42787393520875,
-0.424275166859475,-0.405758519692253,-0.325536566182482,-0.281740120617086,
-0.275267094480029,-0.271364303988575,-0.268340089133171,-0.265538401924824,
-0.261004058170068,-0.248366526641298,-0.22953730751555,-0.193035807796621,
-0.118118298295534,-0.111729377774037,-0.10916430395282,-0.107590514978991,
-0.105855895048481,-0.103355943930342,-0.096903514059749,-0.0634855304692036,
-0.000963188783679523),.UNSPECIFIED.);
#321=B_SPLINE_CURVE_WITH_KNOTS('',3,(#35957,#35958,#35959,#35960,#35961,
#35962,#35963,#35964,#35965,#35966),.UNSPECIFIED.,.F.,.F.,(4,1,1,1,1,1,
1,4),(-154.889187401721,-153.991685902111,-152.99173988976,-151.991793877409,
-150.991847865057,-149.991901852706,-148.991955840354,-148.606018529037),
 .UNSPECIFIED.);
#322=B_SPLINE_CURVE_WITH_KNOTS('',3,(#36691,#36692,#36693,#36694,#36695,
#36696,#36697,#36698,#36699,#36700,#36701,#36702,#36703,#36704),
 .UNSPECIFIED.,.F.,.F.,(4,2,2,2,2,2,4),(0.00555754112882316,0.130635807126562,
0.266975111939351,0.422108165342909,0.562616294044253,0.663795202990439,
0.760829564106722),.UNSPECIFIED.);
#323=B_SPLINE_CURVE_WITH_KNOTS('',3,(#36705,#36706,#36707,#36708,#36709,
#36710,#36711,#36712,#36713,#36714,#36715,#36716,#36717,#36718),
 .UNSPECIFIED.,.F.,.F.,(4,2,2,2,2,2,4),(0.00715775406190771,0.144210143720968,
0.294872793307161,0.424783240858239,0.547591224239104,0.631024462616706,
0.688336229299088),.UNSPECIFIED.);
#392=FACE_BOUND('',#1020,.T.);
#393=FACE_BOUND('',#1022,.T.);
#456=CYLINDRICAL_SURFACE('',#4318,3.933);
#457=CYLINDRICAL_SURFACE('',#4320,3.933);
#458=CYLINDRICAL_SURFACE('',#4322,3.22275);
#459=CYLINDRICAL_SURFACE('',#4324,3.22275);
#460=CYLINDRICAL_SURFACE('',#4325,3.22275);
#461=CYLINDRICAL_SURFACE('',#4327,3.22275);
#462=CYLINDRICAL_SURFACE('',#4329,3.933);
#463=CYLINDRICAL_SURFACE('',#4335,0.5);
#464=CYLINDRICAL_SURFACE('',#4341,0.5);
#465=CYLINDRICAL_SURFACE('',#4347,0.5);
#466=CYLINDRICAL_SURFACE('',#4353,0.5);
#467=CYLINDRICAL_SURFACE('',#4359,0.5);
#468=CYLINDRICAL_SURFACE('',#4365,0.5);
#469=CYLINDRICAL_SURFACE('',#4371,0.5);
#470=CYLINDRICAL_SURFACE('',#4372,8.);
#471=CYLINDRICAL_SURFACE('',#4375,8.);
#472=CYLINDRICAL_SURFACE('',#4381,5.);
#473=CYLINDRICAL_SURFACE('',#4383,5.);
#474=CYLINDRICAL_SURFACE('',#4389,0.5);
#475=CYLINDRICAL_SURFACE('',#4395,0.5);
#476=CYLINDRICAL_SURFACE('',#4400,0.5);
#477=CYLINDRICAL_SURFACE('',#4405,0.5);
#478=CYLINDRICAL_SURFACE('',#4410,0.5);
#479=CYLINDRICAL_SURFACE('',#4415,0.5);
#480=CYLINDRICAL_SURFACE('',#4421,0.5);
#481=CYLINDRICAL_SURFACE('',#4423,5.);
#482=CYLINDRICAL_SURFACE('',#4425,5.);
#483=CYLINDRICAL_SURFACE('',#4427,10.);
#505=TOROIDAL_SURFACE('',#4330,5.5,0.5);
#506=TOROIDAL_SURFACE('',#4337,4.5,0.5);
#507=TOROIDAL_SURFACE('',#4343,7.5,0.5);
#508=TOROIDAL_SURFACE('',#4349,7.5,0.5);
#509=TOROIDAL_SURFACE('',#4355,4.5,0.5);
#510=TOROIDAL_SURFACE('',#4361,5.5,0.5);
#511=TOROIDAL_SURFACE('',#4367,9.5,0.5);
#512=TOROIDAL_SURFACE('',#4384,4.5,0.5);
#513=TOROIDAL_SURFACE('',#4391,5.5,0.5);
#514=TOROIDAL_SURFACE('',#4397,7.5,0.5);
#515=TOROIDAL_SURFACE('',#4402,7.5,0.5);
#516=TOROIDAL_SURFACE('',#4407,5.5,0.5);
#517=TOROIDAL_SURFACE('',#4412,4.5,0.5);
#518=TOROIDAL_SURFACE('',#4417,9.5,0.5);
#573=CIRCLE('',#4319,3.933);
#574=CIRCLE('',#4321,3.933);
#575=CIRCLE('',#4323,3.22275);
#576=CIRCLE('',#4326,3.22275);
#577=CIRCLE('',#4328,3.22275);
#578=CIRCLE('',#4331,0.500000000000007);
#579=CIRCLE('',#4332,5.5);
#580=CIRCLE('',#4333,0.5);
#581=CIRCLE('',#4334,5.);
#582=CIRCLE('',#4336,0.5);
#583=CIRCLE('',#4338,0.5);
#584=CIRCLE('',#4339,5.);
#585=CIRCLE('',#4340,4.5);
#586=CIRCLE('',#4342,0.5);
#587=CIRCLE('',#4344,0.500000000000003);
#588=CIRCLE('',#4345,7.5);
#589=CIRCLE('',#4346,8.);
#590=CIRCLE('',#4348,0.5);
#591=CIRCLE('',#4350,0.500000000000003);
#592=CIRCLE('',#4351,7.5);
#593=CIRCLE('',#4352,8.);
#594=CIRCLE('',#4354,0.5);
#595=CIRCLE('',#4356,0.5);
#596=CIRCLE('',#4357,5.);
#597=CIRCLE('',#4358,4.5);
#598=CIRCLE('',#4360,0.5);
#599=CIRCLE('',#4362,0.5);
#600=CIRCLE('',#4363,5.);
#601=CIRCLE('',#4364,5.5);
#602=CIRCLE('',#4366,0.5);
#603=CIRCLE('',#4368,0.500000000000002);
#604=CIRCLE('',#4369,9.5);
#605=CIRCLE('',#4370,10.);
#606=CIRCLE('',#4373,8.);
#607=CIRCLE('',#4376,8.);
#608=CIRCLE('',#4378,4.5);
#609=CIRCLE('',#4379,5.5);
#610=CIRCLE('',#4385,0.500000000000007);
#611=CIRCLE('',#4386,4.5);
#612=CIRCLE('',#4387,0.5);
#613=CIRCLE('',#4388,5.);
#614=CIRCLE('',#4390,0.5);
#615=CIRCLE('',#4392,0.5);
#616=CIRCLE('',#4393,5.);
#617=CIRCLE('',#4394,5.5);
#618=CIRCLE('',#4396,0.5);
#619=CIRCLE('',#4398,0.500000000000003);
#620=CIRCLE('',#4399,7.5);
#621=CIRCLE('',#4401,0.5);
#622=CIRCLE('',#4403,0.500000000000003);
#623=CIRCLE('',#4404,7.5);
#624=CIRCLE('',#4406,0.5);
#625=CIRCLE('',#4408,0.5);
#626=CIRCLE('',#4409,5.);
#627=CIRCLE('',#4411,0.5);
#628=CIRCLE('',#4413,0.5);
#629=CIRCLE('',#4414,5.);
#630=CIRCLE('',#4416,0.5);
#631=CIRCLE('',#4418,0.500000000000002);
#632=CIRCLE('',#4419,9.5);
#633=CIRCLE('',#4420,10.);
#757=FACE_OUTER_BOUND('',#968,.T.);
#758=FACE_OUTER_BOUND('',#969,.T.);
#759=FACE_OUTER_BOUND('',#970,.T.);
#760=FACE_OUTER_BOUND('',#971,.T.);
#761=FACE_OUTER_BOUND('',#972,.T.);
#762=FACE_OUTER_BOUND('',#973,.T.);
#763=FACE_OUTER_BOUND('',#974,.T.);
#764=FACE_OUTER_BOUND('',#975,.T.);
#765=FACE_OUTER_BOUND('',#976,.T.);
#766=FACE_OUTER_BOUND('',#977,.T.);
#767=FACE_OUTER_BOUND('',#978,.T.);
#768=FACE_OUTER_BOUND('',#979,.T.);
#769=FACE_OUTER_BOUND('',#980,.T.);
#770=FACE_OUTER_BOUND('',#981,.T.);
#771=FACE_OUTER_BOUND('',#982,.T.);
#772=FACE_OUTER_BOUND('',#983,.T.);
#773=FACE_OUTER_BOUND('',#984,.T.);
#774=FACE_OUTER_BOUND('',#985,.T.);
#775=FACE_OUTER_BOUND('',#986,.T.);
#776=FACE_OUTER_BOUND('',#987,.T.);
#777=FACE_OUTER_BOUND('',#988,.T.);
#778=FACE_OUTER_BOUND('',#989,.T.);
#779=FACE_OUTER_BOUND('',#990,.T.);
#780=FACE_OUTER_BOUND('',#991,.T.);
#781=FACE_OUTER_BOUND('',#992,.T.);
#782=FACE_OUTER_BOUND('',#993,.T.);
#783=FACE_OUTER_BOUND('',#994,.T.);
#784=FACE_OUTER_BOUND('',#995,.T.);
#785=FACE_OUTER_BOUND('',#996,.T.);
#786=FACE_OUTER_BOUND('',#997,.T.);
#787=FACE_OUTER_BOUND('',#998,.T.);
#788=FACE_OUTER_BOUND('',#999,.T.);
#789=FACE_OUTER_BOUND('',#1000,.T.);
#790=FACE_OUTER_BOUND('',#1001,.T.);
#791=FACE_OUTER_BOUND('',#1002,.T.);
#792=FACE_OUTER_BOUND('',#1003,.T.);
#793=FACE_OUTER_BOUND('',#1004,.T.);
#794=FACE_OUTER_BOUND('',#1005,.T.);
#795=FACE_OUTER_BOUND('',#1006,.T.);
#796=FACE_OUTER_BOUND('',#1007,.T.);
#797=FACE_OUTER_BOUND('',#1008,.T.);
#798=FACE_OUTER_BOUND('',#1009,.T.);
#799=FACE_OUTER_BOUND('',#1010,.T.);
#800=FACE_OUTER_BOUND('',#1011,.T.);
#801=FACE_OUTER_BOUND('',#1012,.T.);
#802=FACE_OUTER_BOUND('',#1013,.T.);
#803=FACE_OUTER_BOUND('',#1014,.T.);
#804=FACE_OUTER_BOUND('',#1015,.T.);
#805=FACE_OUTER_BOUND('',#1016,.T.);
#806=FACE_OUTER_BOUND('',#1017,.T.);
#807=FACE_OUTER_BOUND('',#1018,.T.);
#808=FACE_OUTER_BOUND('',#1019,.T.);
#809=FACE_OUTER_BOUND('',#1021,.T.);
#968=EDGE_LOOP('',(#3332,#3333,#3334,#3335));
#969=EDGE_LOOP('',(#3336,#3337,#3338,#3339));
#970=EDGE_LOOP('',(#3340,#3341,#3342,#3343,#3344));
#971=EDGE_LOOP('',(#3345,#3346,#3347,#3348,#3349));
#972=EDGE_LOOP('',(#3350,#3351,#3352));
#973=EDGE_LOOP('',(#3353,#3354,#3355,#3356,#3357,#3358,#3359,#3360,#3361,
#3362));
#974=EDGE_LOOP('',(#3363,#3364,#3365,#3366,#3367,#3368));
#975=EDGE_LOOP('',(#3369,#3370,#3371,#3372));
#976=EDGE_LOOP('',(#3373,#3374,#3375,#3376,#3377,#3378,#3379,#3380,#3381,
#3382));
#977=EDGE_LOOP('',(#3383,#3384,#3385,#3386));
#978=EDGE_LOOP('',(#3387,#3388,#3389,#3390));
#979=EDGE_LOOP('',(#3391,#3392,#3393,#3394));
#980=EDGE_LOOP('',(#3395,#3396,#3397,#3398));
#981=EDGE_LOOP('',(#3399,#3400,#3401,#3402));
#982=EDGE_LOOP('',(#3403,#3404,#3405,#3406));
#983=EDGE_LOOP('',(#3407,#3408,#3409,#3410));
#984=EDGE_LOOP('',(#3411,#3412,#3413,#3414));
#985=EDGE_LOOP('',(#3415,#3416,#3417,#3418));
#986=EDGE_LOOP('',(#3419,#3420,#3421,#3422));
#987=EDGE_LOOP('',(#3423,#3424,#3425,#3426));
#988=EDGE_LOOP('',(#3427,#3428,#3429,#3430));
#989=EDGE_LOOP('',(#3431,#3432,#3433,#3434));
#990=EDGE_LOOP('',(#3435,#3436,#3437,#3438));
#991=EDGE_LOOP('',(#3439,#3440,#3441,#3442));
#992=EDGE_LOOP('',(#3443,#3444,#3445,#3446));
#993=EDGE_LOOP('',(#3447,#3448,#3449,#3450));
#994=EDGE_LOOP('',(#3451,#3452,#3453,#3454,#3455,#3456,#3457,#3458,#3459,
#3460,#3461,#3462));
#995=EDGE_LOOP('',(#3463,#3464,#3465,#3466));
#996=EDGE_LOOP('',(#3467,#3468,#3469,#3470));
#997=EDGE_LOOP('',(#3471,#3472,#3473,#3474));
#998=EDGE_LOOP('',(#3475,#3476,#3477,#3478));
#999=EDGE_LOOP('',(#3479,#3480,#3481,#3482));
#1000=EDGE_LOOP('',(#3483,#3484,#3485,#3486));
#1001=EDGE_LOOP('',(#3487,#3488,#3489,#3490));
#1002=EDGE_LOOP('',(#3491,#3492,#3493,#3494));
#1003=EDGE_LOOP('',(#3495,#3496,#3497,#3498));
#1004=EDGE_LOOP('',(#3499,#3500,#3501,#3502));
#1005=EDGE_LOOP('',(#3503,#3504,#3505,#3506));
#1006=EDGE_LOOP('',(#3507,#3508,#3509,#3510));
#1007=EDGE_LOOP('',(#3511,#3512,#3513,#3514));
#1008=EDGE_LOOP('',(#3515,#3516,#3517,#3518));
#1009=EDGE_LOOP('',(#3519,#3520,#3521,#3522));
#1010=EDGE_LOOP('',(#3523,#3524,#3525,#3526));
#1011=EDGE_LOOP('',(#3527,#3528,#3529,#3530));
#1012=EDGE_LOOP('',(#3531,#3532,#3533,#3534));
#1013=EDGE_LOOP('',(#3535,#3536,#3537,#3538));
#1014=EDGE_LOOP('',(#3539,#3540,#3541,#3542));
#1015=EDGE_LOOP('',(#3543,#3544,#3545,#3546));
#1016=EDGE_LOOP('',(#3547,#3548,#3549,#3550));
#1017=EDGE_LOOP('',(#3551,#3552,#3553,#3554,#3555,#3556,#3557,#3558,#3559,
#3560,#3561,#3562));
#1018=EDGE_LOOP('',(#3563,#3564,#3565,#3566));
#1019=EDGE_LOOP('',(#3567,#3568,#3569,#3570,#3571,#3572));
#1020=EDGE_LOOP('',(#3573,#3574,#3575,#3576,#3577));
#1021=EDGE_LOOP('',(#3578,#3579,#3580,#3581,#3582,#3583));
#1022=EDGE_LOOP('',(#3584,#3585,#3586,#3587));
#1185=LINE('',#33624,#1398);
#1186=LINE('',#33879,#1399);
#1187=LINE('',#34272,#1400);
#1188=LINE('',#34413,#1401);
#1189=LINE('',#34715,#1402);
#1190=LINE('',#36732,#1403);
#1191=LINE('',#36733,#1404);
#1192=LINE('',#36744,#1405);
#1193=LINE('',#36745,#1406);
#1194=LINE('',#36756,#1407);
#1195=LINE('',#36757,#1408);
#1196=LINE('',#36768,#1409);
#1197=LINE('',#36769,#1410);
#1198=LINE('',#36780,#1411);
#1199=LINE('',#36781,#1412);
#1200=LINE('',#36792,#1413);
#1201=LINE('',#36793,#1414);
#1202=LINE('',#36801,#1415);
#1203=LINE('',#36802,#1416);
#1204=LINE('',#36805,#1417);
#1205=LINE('',#36808,#1418);
#1206=LINE('',#36811,#1419);
#1207=LINE('',#36812,#1420);
#1208=LINE('',#36815,#1421);
#1209=LINE('',#36819,#1422);
#1210=LINE('',#36821,#1423);
#1211=LINE('',#36825,#1424);
#1212=LINE('',#36828,#1425);
#1213=LINE('',#36830,#1426);
#1214=LINE('',#36832,#1427);
#1215=LINE('',#36833,#1428);
#1216=LINE('',#36835,#1429);
#1217=LINE('',#36850,#1430);
#1218=LINE('',#36851,#1431);
#1219=LINE('',#36861,#1432);
#1220=LINE('',#36862,#1433);
#1221=LINE('',#36870,#1434);
#1222=LINE('',#36878,#1435);
#1223=LINE('',#36886,#1436);
#1224=LINE('',#36894,#1437);
#1225=LINE('',#36902,#1438);
#1226=LINE('',#36903,#1439);
#1227=LINE('',#36905,#1440);
#1228=LINE('',#36907,#1441);
#1229=LINE('',#36908,#1442);
#1230=LINE('',#36910,#1443);
#1231=LINE('',#36913,#1444);
#1398=VECTOR('',#4958,3.933);
#1399=VECTOR('',#4963,3.933);
#1400=VECTOR('',#4968,3.22275);
#1401=VECTOR('',#4973,3.22275);
#1402=VECTOR('',#4976,3.22275);
#1403=VECTOR('',#4999,10.);
#1404=VECTOR('',#5000,10.);
#1405=VECTOR('',#5013,10.);
#1406=VECTOR('',#5014,10.);
#1407=VECTOR('',#5027,10.);
#1408=VECTOR('',#5028,10.);
#1409=VECTOR('',#5041,10.);
#1410=VECTOR('',#5042,10.);
#1411=VECTOR('',#5055,10.);
#1412=VECTOR('',#5056,10.);
#1413=VECTOR('',#5069,10.);
#1414=VECTOR('',#5070,10.);
#1415=VECTOR('',#5081,10.);
#1416=VECTOR('',#5082,10.);
#1417=VECTOR('',#5085,10.);
#1418=VECTOR('',#5088,10.);
#1419=VECTOR('',#5091,10.);
#1420=VECTOR('',#5092,10.);
#1421=VECTOR('',#5095,10.);
#1422=VECTOR('',#5100,10.);
#1423=VECTOR('',#5101,10.);
#1424=VECTOR('',#5104,10.);
#1425=VECTOR('',#5107,10.);
#1426=VECTOR('',#5110,10.);
#1427=VECTOR('',#5113,10.);
#1428=VECTOR('',#5114,10.);
#1429=VECTOR('',#5117,10.);
#1430=VECTOR('',#5134,10.);
#1431=VECTOR('',#5135,10.);
#1432=VECTOR('',#5148,10.);
#1433=VECTOR('',#5149,10.);
#1434=VECTOR('',#5160,10.);
#1435=VECTOR('',#5171,10.);
#1436=VECTOR('',#5182,10.);
#1437=VECTOR('',#5193,10.);
#1438=VECTOR('',#5204,10.);
#1439=VECTOR('',#5205,10.);
#1440=VECTOR('',#5208,10.);
#1441=VECTOR('',#5211,10.);
#1442=VECTOR('',#5212,10.);
#1443=VECTOR('',#5215,10.);
#1444=VECTOR('',#5220,10.);
#1775=VERTEX_POINT('',#33622);
#1776=VERTEX_POINT('',#33623);
#1777=VERTEX_POINT('',#33625);
#1778=VERTEX_POINT('',#33732);
#1779=VERTEX_POINT('',#33877);
#1780=VERTEX_POINT('',#33878);
#1781=VERTEX_POINT('',#33880);
#1782=VERTEX_POINT('',#34056);
#1783=VERTEX_POINT('',#34270);
#1784=VERTEX_POINT('',#34271);
#1785=VERTEX_POINT('',#34273);
#1786=VERTEX_POINT('',#34279);
#1787=VERTEX_POINT('',#34281);
#1788=VERTEX_POINT('',#34411);
#1789=VERTEX_POINT('',#34412);
#1790=VERTEX_POINT('',#34414);
#1791=VERTEX_POINT('',#34713);
#1792=VERTEX_POINT('',#34714);
#1793=VERTEX_POINT('',#34716);
#1794=VERTEX_POINT('',#35731);
#1795=VERTEX_POINT('',#35896);
#1796=VERTEX_POINT('',#36720);
#1797=VERTEX_POINT('',#36721);
#1798=VERTEX_POINT('',#36723);
#1799=VERTEX_POINT('',#36725);
#1800=VERTEX_POINT('',#36729);
#1801=VERTEX_POINT('',#36730);
#1802=VERTEX_POINT('',#36735);
#1803=VERTEX_POINT('',#36736);
#1804=VERTEX_POINT('',#36741);
#1805=VERTEX_POINT('',#36742);
#1806=VERTEX_POINT('',#36747);
#1807=VERTEX_POINT('',#36748);
#1808=VERTEX_POINT('',#36753);
#1809=VERTEX_POINT('',#36754);
#1810=VERTEX_POINT('',#36759);
#1811=VERTEX_POINT('',#36760);
#1812=VERTEX_POINT('',#36765);
#1813=VERTEX_POINT('',#36766);
#1814=VERTEX_POINT('',#36771);
#1815=VERTEX_POINT('',#36772);
#1816=VERTEX_POINT('',#36777);
#1817=VERTEX_POINT('',#36778);
#1818=VERTEX_POINT('',#36783);
#1819=VERTEX_POINT('',#36784);
#1820=VERTEX_POINT('',#36789);
#1821=VERTEX_POINT('',#36790);
#1822=VERTEX_POINT('',#36795);
#1823=VERTEX_POINT('',#36796);
#1824=VERTEX_POINT('',#36804);
#1825=VERTEX_POINT('',#36806);
#1826=VERTEX_POINT('',#36810);
#1827=VERTEX_POINT('',#36814);
#1828=VERTEX_POINT('',#36818);
#1829=VERTEX_POINT('',#36820);
#1830=VERTEX_POINT('',#36822);
#1831=VERTEX_POINT('',#36824);
#1832=VERTEX_POINT('',#36826);
#1833=VERTEX_POINT('',#36838);
#1834=VERTEX_POINT('',#36839);
#1835=VERTEX_POINT('',#36841);
#1836=VERTEX_POINT('',#36843);
#1837=VERTEX_POINT('',#36847);
#1838=VERTEX_POINT('',#36848);
#1839=VERTEX_POINT('',#36853);
#1840=VERTEX_POINT('',#36854);
#1841=VERTEX_POINT('',#36859);
#1842=VERTEX_POINT('',#36864);
#1843=VERTEX_POINT('',#36868);
#1844=VERTEX_POINT('',#36872);
#1845=VERTEX_POINT('',#36876);
#1846=VERTEX_POINT('',#36880);
#1847=VERTEX_POINT('',#36884);
#1848=VERTEX_POINT('',#36888);
#1849=VERTEX_POINT('',#36892);
#1850=VERTEX_POINT('',#36896);
#1851=VERTEX_POINT('',#36897);
#2317=EDGE_CURVE('',#1775,#1776,#1185,.T.);
#2318=EDGE_CURVE('',#1777,#1776,#304,.T.);
#2319=EDGE_CURVE('',#1778,#1777,#573,.T.);
#2320=EDGE_CURVE('',#1775,#1778,#305,.T.);
#2321=EDGE_CURVE('',#1779,#1780,#1186,.T.);
#2322=EDGE_CURVE('',#1781,#1779,#306,.T.);
#2323=EDGE_CURVE('',#1782,#1781,#574,.T.);
#2324=EDGE_CURVE('',#1780,#1782,#307,.T.);
#2325=EDGE_CURVE('',#1783,#1784,#1187,.T.);
#2326=EDGE_CURVE('',#1784,#1785,#308,.T.);
#2327=EDGE_CURVE('',#1786,#1785,#575,.T.);
#2328=EDGE_CURVE('',#1787,#1786,#309,.T.);
#2329=EDGE_CURVE('',#1783,#1787,#310,.T.);
#2330=EDGE_CURVE('',#1788,#1789,#1188,.T.);
#2331=EDGE_CURVE('',#1789,#1790,#311,.F.);
#2332=EDGE_CURVE('',#1790,#1784,#312,.T.);
#2333=EDGE_CURVE('',#1788,#1783,#313,.T.);
#2334=EDGE_CURVE('',#1791,#1792,#1189,.T.);
#2335=EDGE_CURVE('',#1793,#1791,#576,.T.);
#2336=EDGE_CURVE('',#1793,#1792,#314,.F.);
#2337=EDGE_CURVE('',#1781,#1793,#315,.T.);
#2338=EDGE_CURVE('',#1779,#1775,#316,.T.);
#2339=EDGE_CURVE('',#1785,#1778,#317,.T.);
#2340=EDGE_CURVE('',#1792,#1789,#318,.F.);
#2341=EDGE_CURVE('',#1794,#1788,#319,.T.);
#2342=EDGE_CURVE('',#1795,#1794,#320,.T.);
#2343=EDGE_CURVE('',#1791,#1795,#577,.T.);
#2344=EDGE_CURVE('',#1776,#1780,#321,.T.);
#2345=EDGE_CURVE('',#1795,#1782,#322,.T.);
#2346=EDGE_CURVE('',#1777,#1786,#323,.T.);
#2347=EDGE_CURVE('',#1796,#1797,#578,.T.);
#2348=EDGE_CURVE('',#1797,#1798,#579,.T.);
#2349=EDGE_CURVE('',#1798,#1799,#580,.T.);
#2350=EDGE_CURVE('',#1799,#1796,#581,.T.);
#2351=EDGE_CURVE('',#1800,#1801,#582,.T.);
#2352=EDGE_CURVE('',#1801,#1799,#1190,.T.);
#2353=EDGE_CURVE('',#1798,#1800,#1191,.T.);
#2354=EDGE_CURVE('',#1802,#1803,#583,.T.);
#2355=EDGE_CURVE('',#1803,#1801,#584,.T.);
#2356=EDGE_CURVE('',#1800,#1802,#585,.T.);
#2357=EDGE_CURVE('',#1804,#1805,#586,.T.);
#2358=EDGE_CURVE('',#1805,#1803,#1192,.T.);
#2359=EDGE_CURVE('',#1802,#1804,#1193,.T.);
#2360=EDGE_CURVE('',#1806,#1807,#587,.T.);
#2361=EDGE_CURVE('',#1807,#1805,#588,.T.);
#2362=EDGE_CURVE('',#1804,#1806,#589,.T.);
#2363=EDGE_CURVE('',#1808,#1809,#590,.T.);
#2364=EDGE_CURVE('',#1809,#1807,#1194,.T.);
#2365=EDGE_CURVE('',#1806,#1808,#1195,.T.);
#2366=EDGE_CURVE('',#1810,#1811,#591,.T.);
#2367=EDGE_CURVE('',#1811,#1809,#592,.T.);
#2368=EDGE_CURVE('',#1808,#1810,#593,.T.);
#2369=EDGE_CURVE('',#1812,#1813,#594,.T.);
#2370=EDGE_CURVE('',#1813,#1811,#1196,.T.);
#2371=EDGE_CURVE('',#1810,#1812,#1197,.T.);
#2372=EDGE_CURVE('',#1814,#1815,#595,.T.);
#2373=EDGE_CURVE('',#1815,#1813,#596,.T.);
#2374=EDGE_CURVE('',#1812,#1814,#597,.T.);
#2375=EDGE_CURVE('',#1816,#1817,#598,.T.);
#2376=EDGE_CURVE('',#1817,#1815,#1198,.T.);
#2377=EDGE_CURVE('',#1814,#1816,#1199,.T.);
#2378=EDGE_CURVE('',#1818,#1819,#599,.T.);
#2379=EDGE_CURVE('',#1819,#1817,#600,.T.);
#2380=EDGE_CURVE('',#1816,#1818,#601,.T.);
#2381=EDGE_CURVE('',#1820,#1821,#602,.T.);
#2382=EDGE_CURVE('',#1821,#1819,#1200,.T.);
#2383=EDGE_CURVE('',#1818,#1820,#1201,.T.);
#2384=EDGE_CURVE('',#1822,#1823,#603,.T.);
#2385=EDGE_CURVE('',#1823,#1821,#604,.T.);
#2386=EDGE_CURVE('',#1820,#1822,#605,.T.);
#2387=EDGE_CURVE('',#1822,#1797,#1202,.T.);
#2388=EDGE_CURVE('',#1796,#1823,#1203,.T.);
#2389=EDGE_CURVE('',#1808,#1824,#1204,.T.);
#2390=EDGE_CURVE('',#1825,#1824,#606,.T.);
#2391=EDGE_CURVE('',#1825,#1810,#1205,.T.);
#2392=EDGE_CURVE('',#1826,#1806,#1206,.T.);
#2393=EDGE_CURVE('',#1824,#1826,#1207,.T.);
#2394=EDGE_CURVE('',#1804,#1827,#1208,.T.);
#2395=EDGE_CURVE('',#1826,#1827,#607,.T.);
#2396=EDGE_CURVE('',#1828,#1822,#1209,.T.);
#2397=EDGE_CURVE('',#1829,#1828,#1210,.T.);
#2398=EDGE_CURVE('',#1830,#1829,#608,.T.);
#2399=EDGE_CURVE('',#1831,#1830,#1211,.T.);
#2400=EDGE_CURVE('',#1832,#1831,#609,.T.);
#2401=EDGE_CURVE('',#1827,#1832,#1212,.T.);
#2402=EDGE_CURVE('',#1819,#1796,#1213,.T.);
#2403=EDGE_CURVE('',#1815,#1801,#1214,.T.);
#2404=EDGE_CURVE('',#1803,#1813,#1215,.T.);
#2405=EDGE_CURVE('',#1799,#1817,#1216,.T.);
#2406=EDGE_CURVE('',#1833,#1834,#610,.T.);
#2407=EDGE_CURVE('',#1834,#1835,#611,.T.);
#2408=EDGE_CURVE('',#1835,#1836,#612,.T.);
#2409=EDGE_CURVE('',#1836,#1833,#613,.T.);
#2410=EDGE_CURVE('',#1837,#1838,#614,.T.);
#2411=EDGE_CURVE('',#1838,#1836,#1217,.T.);
#2412=EDGE_CURVE('',#1835,#1837,#1218,.T.);
#2413=EDGE_CURVE('',#1839,#1840,#615,.T.);
#2414=EDGE_CURVE('',#1840,#1838,#616,.T.);
#2415=EDGE_CURVE('',#1837,#1839,#617,.T.);
#2416=EDGE_CURVE('',#1825,#1841,#618,.T.);
#2417=EDGE_CURVE('',#1841,#1840,#1219,.T.);
#2418=EDGE_CURVE('',#1839,#1825,#1220,.T.);
#2419=EDGE_CURVE('',#1824,#1842,#619,.T.);
#2420=EDGE_CURVE('',#1842,#1841,#620,.T.);
#2421=EDGE_CURVE('',#1826,#1843,#621,.T.);
#2422=EDGE_CURVE('',#1843,#1842,#1221,.T.);
#2423=EDGE_CURVE('',#1827,#1844,#622,.T.);
#2424=EDGE_CURVE('',#1844,#1843,#623,.T.);
#2425=EDGE_CURVE('',#1832,#1845,#624,.T.);
#2426=EDGE_CURVE('',#1845,#1844,#1222,.T.);
#2427=EDGE_CURVE('',#1831,#1846,#625,.T.);
#2428=EDGE_CURVE('',#1846,#1845,#626,.T.);
#2429=EDGE_CURVE('',#1830,#1847,#627,.T.);
#2430=EDGE_CURVE('',#1847,#1846,#1223,.T.);
#2431=EDGE_CURVE('',#1829,#1848,#628,.T.);
#2432=EDGE_CURVE('',#1848,#1847,#629,.T.);
#2433=EDGE_CURVE('',#1828,#1849,#630,.T.);
#2434=EDGE_CURVE('',#1849,#1848,#1224,.T.);
#2435=EDGE_CURVE('',#1850,#1851,#631,.T.);
#2436=EDGE_CURVE('',#1851,#1849,#632,.T.);
#2437=EDGE_CURVE('',#1828,#1850,#633,.T.);
#2438=EDGE_CURVE('',#1850,#1834,#1225,.T.);
#2439=EDGE_CURVE('',#1833,#1851,#1226,.T.);
#2440=EDGE_CURVE('',#1848,#1833,#1227,.T.);
#2441=EDGE_CURVE('',#1846,#1838,#1228,.T.);
#2442=EDGE_CURVE('',#1840,#1845,#1229,.T.);
#2443=EDGE_CURVE('',#1836,#1847,#1230,.T.);
#2444=EDGE_CURVE('',#1820,#1850,#1231,.T.);
#3332=ORIENTED_EDGE('',*,*,#2317,.T.);
#3333=ORIENTED_EDGE('',*,*,#2318,.F.);
#3334=ORIENTED_EDGE('',*,*,#2319,.F.);
#3335=ORIENTED_EDGE('',*,*,#2320,.F.);
#3336=ORIENTED_EDGE('',*,*,#2321,.F.);
#3337=ORIENTED_EDGE('',*,*,#2322,.F.);
#3338=ORIENTED_EDGE('',*,*,#2323,.F.);
#3339=ORIENTED_EDGE('',*,*,#2324,.F.);
#3340=ORIENTED_EDGE('',*,*,#2325,.T.);
#3341=ORIENTED_EDGE('',*,*,#2326,.T.);
#3342=ORIENTED_EDGE('',*,*,#2327,.F.);
#3343=ORIENTED_EDGE('',*,*,#2328,.F.);
#3344=ORIENTED_EDGE('',*,*,#2329,.F.);
#3345=ORIENTED_EDGE('',*,*,#2330,.T.);
#3346=ORIENTED_EDGE('',*,*,#2331,.T.);
#3347=ORIENTED_EDGE('',*,*,#2332,.T.);
#3348=ORIENTED_EDGE('',*,*,#2325,.F.);
#3349=ORIENTED_EDGE('',*,*,#2333,.F.);
#3350=ORIENTED_EDGE('',*,*,#2334,.F.);
#3351=ORIENTED_EDGE('',*,*,#2335,.F.);
#3352=ORIENTED_EDGE('',*,*,#2336,.T.);
#3353=ORIENTED_EDGE('',*,*,#2337,.F.);
#3354=ORIENTED_EDGE('',*,*,#2322,.T.);
#3355=ORIENTED_EDGE('',*,*,#2338,.T.);
#3356=ORIENTED_EDGE('',*,*,#2320,.T.);
#3357=ORIENTED_EDGE('',*,*,#2339,.F.);
#3358=ORIENTED_EDGE('',*,*,#2326,.F.);
#3359=ORIENTED_EDGE('',*,*,#2332,.F.);
#3360=ORIENTED_EDGE('',*,*,#2331,.F.);
#3361=ORIENTED_EDGE('',*,*,#2340,.F.);
#3362=ORIENTED_EDGE('',*,*,#2336,.F.);
#3363=ORIENTED_EDGE('',*,*,#2334,.T.);
#3364=ORIENTED_EDGE('',*,*,#2340,.T.);
#3365=ORIENTED_EDGE('',*,*,#2330,.F.);
#3366=ORIENTED_EDGE('',*,*,#2341,.F.);
#3367=ORIENTED_EDGE('',*,*,#2342,.F.);
#3368=ORIENTED_EDGE('',*,*,#2343,.F.);
#3369=ORIENTED_EDGE('',*,*,#2321,.T.);
#3370=ORIENTED_EDGE('',*,*,#2344,.F.);
#3371=ORIENTED_EDGE('',*,*,#2317,.F.);
#3372=ORIENTED_EDGE('',*,*,#2338,.F.);
#3373=ORIENTED_EDGE('',*,*,#2345,.F.);
#3374=ORIENTED_EDGE('',*,*,#2342,.T.);
#3375=ORIENTED_EDGE('',*,*,#2341,.T.);
#3376=ORIENTED_EDGE('',*,*,#2333,.T.);
#3377=ORIENTED_EDGE('',*,*,#2329,.T.);
#3378=ORIENTED_EDGE('',*,*,#2328,.T.);
#3379=ORIENTED_EDGE('',*,*,#2346,.F.);
#3380=ORIENTED_EDGE('',*,*,#2318,.T.);
#3381=ORIENTED_EDGE('',*,*,#2344,.T.);
#3382=ORIENTED_EDGE('',*,*,#2324,.T.);
#3383=ORIENTED_EDGE('',*,*,#2347,.T.);
#3384=ORIENTED_EDGE('',*,*,#2348,.T.);
#3385=ORIENTED_EDGE('',*,*,#2349,.T.);
#3386=ORIENTED_EDGE('',*,*,#2350,.T.);
#3387=ORIENTED_EDGE('',*,*,#2351,.T.);
#3388=ORIENTED_EDGE('',*,*,#2352,.T.);
#3389=ORIENTED_EDGE('',*,*,#2349,.F.);
#3390=ORIENTED_EDGE('',*,*,#2353,.T.);
#3391=ORIENTED_EDGE('',*,*,#2354,.T.);
#3392=ORIENTED_EDGE('',*,*,#2355,.T.);
#3393=ORIENTED_EDGE('',*,*,#2351,.F.);
#3394=ORIENTED_EDGE('',*,*,#2356,.T.);
#3395=ORIENTED_EDGE('',*,*,#2357,.T.);
#3396=ORIENTED_EDGE('',*,*,#2358,.T.);
#3397=ORIENTED_EDGE('',*,*,#2354,.F.);
#3398=ORIENTED_EDGE('',*,*,#2359,.T.);
#3399=ORIENTED_EDGE('',*,*,#2360,.T.);
#3400=ORIENTED_EDGE('',*,*,#2361,.T.);
#3401=ORIENTED_EDGE('',*,*,#2357,.F.);
#3402=ORIENTED_EDGE('',*,*,#2362,.T.);
#3403=ORIENTED_EDGE('',*,*,#2363,.T.);
#3404=ORIENTED_EDGE('',*,*,#2364,.T.);
#3405=ORIENTED_EDGE('',*,*,#2360,.F.);
#3406=ORIENTED_EDGE('',*,*,#2365,.T.);
#3407=ORIENTED_EDGE('',*,*,#2366,.T.);
#3408=ORIENTED_EDGE('',*,*,#2367,.T.);
#3409=ORIENTED_EDGE('',*,*,#2363,.F.);
#3410=ORIENTED_EDGE('',*,*,#2368,.T.);
#3411=ORIENTED_EDGE('',*,*,#2369,.T.);
#3412=ORIENTED_EDGE('',*,*,#2370,.T.);
#3413=ORIENTED_EDGE('',*,*,#2366,.F.);
#3414=ORIENTED_EDGE('',*,*,#2371,.T.);
#3415=ORIENTED_EDGE('',*,*,#2372,.T.);
#3416=ORIENTED_EDGE('',*,*,#2373,.T.);
#3417=ORIENTED_EDGE('',*,*,#2369,.F.);
#3418=ORIENTED_EDGE('',*,*,#2374,.T.);
#3419=ORIENTED_EDGE('',*,*,#2375,.T.);
#3420=ORIENTED_EDGE('',*,*,#2376,.T.);
#3421=ORIENTED_EDGE('',*,*,#2372,.F.);
#3422=ORIENTED_EDGE('',*,*,#2377,.T.);
#3423=ORIENTED_EDGE('',*,*,#2378,.T.);
#3424=ORIENTED_EDGE('',*,*,#2379,.T.);
#3425=ORIENTED_EDGE('',*,*,#2375,.F.);
#3426=ORIENTED_EDGE('',*,*,#2380,.T.);
#3427=ORIENTED_EDGE('',*,*,#2381,.T.);
#3428=ORIENTED_EDGE('',*,*,#2382,.T.);
#3429=ORIENTED_EDGE('',*,*,#2378,.F.);
#3430=ORIENTED_EDGE('',*,*,#2383,.T.);
#3431=ORIENTED_EDGE('',*,*,#2384,.T.);
#3432=ORIENTED_EDGE('',*,*,#2385,.T.);
#3433=ORIENTED_EDGE('',*,*,#2381,.F.);
#3434=ORIENTED_EDGE('',*,*,#2386,.T.);
#3435=ORIENTED_EDGE('',*,*,#2384,.F.);
#3436=ORIENTED_EDGE('',*,*,#2387,.T.);
#3437=ORIENTED_EDGE('',*,*,#2347,.F.);
#3438=ORIENTED_EDGE('',*,*,#2388,.T.);
#3439=ORIENTED_EDGE('',*,*,#2368,.F.);
#3440=ORIENTED_EDGE('',*,*,#2389,.T.);
#3441=ORIENTED_EDGE('',*,*,#2390,.F.);
#3442=ORIENTED_EDGE('',*,*,#2391,.T.);
#3443=ORIENTED_EDGE('',*,*,#2365,.F.);
#3444=ORIENTED_EDGE('',*,*,#2392,.F.);
#3445=ORIENTED_EDGE('',*,*,#2393,.F.);
#3446=ORIENTED_EDGE('',*,*,#2389,.F.);
#3447=ORIENTED_EDGE('',*,*,#2362,.F.);
#3448=ORIENTED_EDGE('',*,*,#2394,.T.);
#3449=ORIENTED_EDGE('',*,*,#2395,.F.);
#3450=ORIENTED_EDGE('',*,*,#2392,.T.);
#3451=ORIENTED_EDGE('',*,*,#2359,.F.);
#3452=ORIENTED_EDGE('',*,*,#2356,.F.);
#3453=ORIENTED_EDGE('',*,*,#2353,.F.);
#3454=ORIENTED_EDGE('',*,*,#2348,.F.);
#3455=ORIENTED_EDGE('',*,*,#2387,.F.);
#3456=ORIENTED_EDGE('',*,*,#2396,.F.);
#3457=ORIENTED_EDGE('',*,*,#2397,.F.);
#3458=ORIENTED_EDGE('',*,*,#2398,.F.);
#3459=ORIENTED_EDGE('',*,*,#2399,.F.);
#3460=ORIENTED_EDGE('',*,*,#2400,.F.);
#3461=ORIENTED_EDGE('',*,*,#2401,.F.);
#3462=ORIENTED_EDGE('',*,*,#2394,.F.);
#3463=ORIENTED_EDGE('',*,*,#2382,.F.);
#3464=ORIENTED_EDGE('',*,*,#2385,.F.);
#3465=ORIENTED_EDGE('',*,*,#2388,.F.);
#3466=ORIENTED_EDGE('',*,*,#2402,.F.);
#3467=ORIENTED_EDGE('',*,*,#2373,.F.);
#3468=ORIENTED_EDGE('',*,*,#2403,.T.);
#3469=ORIENTED_EDGE('',*,*,#2355,.F.);
#3470=ORIENTED_EDGE('',*,*,#2404,.T.);
#3471=ORIENTED_EDGE('',*,*,#2376,.F.);
#3472=ORIENTED_EDGE('',*,*,#2405,.F.);
#3473=ORIENTED_EDGE('',*,*,#2352,.F.);
#3474=ORIENTED_EDGE('',*,*,#2403,.F.);
#3475=ORIENTED_EDGE('',*,*,#2379,.F.);
#3476=ORIENTED_EDGE('',*,*,#2402,.T.);
#3477=ORIENTED_EDGE('',*,*,#2350,.F.);
#3478=ORIENTED_EDGE('',*,*,#2405,.T.);
#3479=ORIENTED_EDGE('',*,*,#2406,.T.);
#3480=ORIENTED_EDGE('',*,*,#2407,.T.);
#3481=ORIENTED_EDGE('',*,*,#2408,.T.);
#3482=ORIENTED_EDGE('',*,*,#2409,.T.);
#3483=ORIENTED_EDGE('',*,*,#2410,.T.);
#3484=ORIENTED_EDGE('',*,*,#2411,.T.);
#3485=ORIENTED_EDGE('',*,*,#2408,.F.);
#3486=ORIENTED_EDGE('',*,*,#2412,.T.);
#3487=ORIENTED_EDGE('',*,*,#2413,.T.);
#3488=ORIENTED_EDGE('',*,*,#2414,.T.);
#3489=ORIENTED_EDGE('',*,*,#2410,.F.);
#3490=ORIENTED_EDGE('',*,*,#2415,.T.);
#3491=ORIENTED_EDGE('',*,*,#2416,.T.);
#3492=ORIENTED_EDGE('',*,*,#2417,.T.);
#3493=ORIENTED_EDGE('',*,*,#2413,.F.);
#3494=ORIENTED_EDGE('',*,*,#2418,.T.);
#3495=ORIENTED_EDGE('',*,*,#2419,.T.);
#3496=ORIENTED_EDGE('',*,*,#2420,.T.);
#3497=ORIENTED_EDGE('',*,*,#2416,.F.);
#3498=ORIENTED_EDGE('',*,*,#2390,.T.);
#3499=ORIENTED_EDGE('',*,*,#2421,.T.);
#3500=ORIENTED_EDGE('',*,*,#2422,.T.);
#3501=ORIENTED_EDGE('',*,*,#2419,.F.);
#3502=ORIENTED_EDGE('',*,*,#2393,.T.);
#3503=ORIENTED_EDGE('',*,*,#2423,.T.);
#3504=ORIENTED_EDGE('',*,*,#2424,.T.);
#3505=ORIENTED_EDGE('',*,*,#2421,.F.);
#3506=ORIENTED_EDGE('',*,*,#2395,.T.);
#3507=ORIENTED_EDGE('',*,*,#2425,.T.);
#3508=ORIENTED_EDGE('',*,*,#2426,.T.);
#3509=ORIENTED_EDGE('',*,*,#2423,.F.);
#3510=ORIENTED_EDGE('',*,*,#2401,.T.);
#3511=ORIENTED_EDGE('',*,*,#2427,.T.);
#3512=ORIENTED_EDGE('',*,*,#2428,.T.);
#3513=ORIENTED_EDGE('',*,*,#2425,.F.);
#3514=ORIENTED_EDGE('',*,*,#2400,.T.);
#3515=ORIENTED_EDGE('',*,*,#2429,.T.);
#3516=ORIENTED_EDGE('',*,*,#2430,.T.);
#3517=ORIENTED_EDGE('',*,*,#2427,.F.);
#3518=ORIENTED_EDGE('',*,*,#2399,.T.);
#3519=ORIENTED_EDGE('',*,*,#2431,.T.);
#3520=ORIENTED_EDGE('',*,*,#2432,.T.);
#3521=ORIENTED_EDGE('',*,*,#2429,.F.);
#3522=ORIENTED_EDGE('',*,*,#2398,.T.);
#3523=ORIENTED_EDGE('',*,*,#2433,.T.);
#3524=ORIENTED_EDGE('',*,*,#2434,.T.);
#3525=ORIENTED_EDGE('',*,*,#2431,.F.);
#3526=ORIENTED_EDGE('',*,*,#2397,.T.);
#3527=ORIENTED_EDGE('',*,*,#2435,.T.);
#3528=ORIENTED_EDGE('',*,*,#2436,.T.);
#3529=ORIENTED_EDGE('',*,*,#2433,.F.);
#3530=ORIENTED_EDGE('',*,*,#2437,.T.);
#3531=ORIENTED_EDGE('',*,*,#2435,.F.);
#3532=ORIENTED_EDGE('',*,*,#2438,.T.);
#3533=ORIENTED_EDGE('',*,*,#2406,.F.);
#3534=ORIENTED_EDGE('',*,*,#2439,.T.);
#3535=ORIENTED_EDGE('',*,*,#2434,.F.);
#3536=ORIENTED_EDGE('',*,*,#2436,.F.);
#3537=ORIENTED_EDGE('',*,*,#2439,.F.);
#3538=ORIENTED_EDGE('',*,*,#2440,.F.);
#3539=ORIENTED_EDGE('',*,*,#2428,.F.);
#3540=ORIENTED_EDGE('',*,*,#2441,.T.);
#3541=ORIENTED_EDGE('',*,*,#2414,.F.);
#3542=ORIENTED_EDGE('',*,*,#2442,.T.);
#3543=ORIENTED_EDGE('',*,*,#2430,.F.);
#3544=ORIENTED_EDGE('',*,*,#2443,.F.);
#3545=ORIENTED_EDGE('',*,*,#2411,.F.);
#3546=ORIENTED_EDGE('',*,*,#2441,.F.);
#3547=ORIENTED_EDGE('',*,*,#2432,.F.);
#3548=ORIENTED_EDGE('',*,*,#2440,.T.);
#3549=ORIENTED_EDGE('',*,*,#2409,.F.);
#3550=ORIENTED_EDGE('',*,*,#2443,.T.);
#3551=ORIENTED_EDGE('',*,*,#2371,.F.);
#3552=ORIENTED_EDGE('',*,*,#2391,.F.);
#3553=ORIENTED_EDGE('',*,*,#2418,.F.);
#3554=ORIENTED_EDGE('',*,*,#2415,.F.);
#3555=ORIENTED_EDGE('',*,*,#2412,.F.);
#3556=ORIENTED_EDGE('',*,*,#2407,.F.);
#3557=ORIENTED_EDGE('',*,*,#2438,.F.);
#3558=ORIENTED_EDGE('',*,*,#2444,.F.);
#3559=ORIENTED_EDGE('',*,*,#2383,.F.);
#3560=ORIENTED_EDGE('',*,*,#2380,.F.);
#3561=ORIENTED_EDGE('',*,*,#2377,.F.);
#3562=ORIENTED_EDGE('',*,*,#2374,.F.);
#3563=ORIENTED_EDGE('',*,*,#2386,.F.);
#3564=ORIENTED_EDGE('',*,*,#2444,.T.);
#3565=ORIENTED_EDGE('',*,*,#2437,.F.);
#3566=ORIENTED_EDGE('',*,*,#2396,.T.);
#3567=ORIENTED_EDGE('',*,*,#2370,.F.);
#3568=ORIENTED_EDGE('',*,*,#2404,.F.);
#3569=ORIENTED_EDGE('',*,*,#2358,.F.);
#3570=ORIENTED_EDGE('',*,*,#2361,.F.);
#3571=ORIENTED_EDGE('',*,*,#2364,.F.);
#3572=ORIENTED_EDGE('',*,*,#2367,.F.);
#3573=ORIENTED_EDGE('',*,*,#2345,.T.);
#3574=ORIENTED_EDGE('',*,*,#2323,.T.);
#3575=ORIENTED_EDGE('',*,*,#2337,.T.);
#3576=ORIENTED_EDGE('',*,*,#2335,.T.);
#3577=ORIENTED_EDGE('',*,*,#2343,.T.);
#3578=ORIENTED_EDGE('',*,*,#2426,.F.);
#3579=ORIENTED_EDGE('',*,*,#2442,.F.);
#3580=ORIENTED_EDGE('',*,*,#2417,.F.);
#3581=ORIENTED_EDGE('',*,*,#2420,.F.);
#3582=ORIENTED_EDGE('',*,*,#2422,.F.);
#3583=ORIENTED_EDGE('',*,*,#2424,.F.);
#3584=ORIENTED_EDGE('',*,*,#2346,.T.);
#3585=ORIENTED_EDGE('',*,*,#2327,.T.);
#3586=ORIENTED_EDGE('',*,*,#2339,.T.);
#3587=ORIENTED_EDGE('',*,*,#2319,.T.);
#3817=PLANE('',#4374);
#3818=PLANE('',#4377);
#3819=PLANE('',#4380);
#3820=PLANE('',#4382);
#3821=PLANE('',#4422);
#3822=PLANE('',#4424);
#3823=PLANE('',#4426);
#3824=PLANE('',#4428);
#3825=PLANE('',#4429);
#3953=ADVANCED_FACE('',(#757),#456,.F.);
#3954=ADVANCED_FACE('',(#758),#457,.F.);
#3955=ADVANCED_FACE('',(#759),#458,.F.);
#3956=ADVANCED_FACE('',(#760),#459,.F.);
#3957=ADVANCED_FACE('',(#761),#460,.F.);
#3958=ADVANCED_FACE('',(#762),#90,.T.);
#3959=ADVANCED_FACE('',(#763),#461,.F.);
#3960=ADVANCED_FACE('',(#764),#462,.F.);
#3961=ADVANCED_FACE('',(#765),#91,.T.);
#3962=ADVANCED_FACE('',(#766),#505,.T.);
#3963=ADVANCED_FACE('',(#767),#463,.T.);
#3964=ADVANCED_FACE('',(#768),#506,.T.);
#3965=ADVANCED_FACE('',(#769),#464,.T.);
#3966=ADVANCED_FACE('',(#770),#507,.T.);
#3967=ADVANCED_FACE('',(#771),#465,.T.);
#3968=ADVANCED_FACE('',(#772),#508,.T.);
#3969=ADVANCED_FACE('',(#773),#466,.T.);
#3970=ADVANCED_FACE('',(#774),#509,.T.);
#3971=ADVANCED_FACE('',(#775),#467,.T.);
#3972=ADVANCED_FACE('',(#776),#510,.T.);
#3973=ADVANCED_FACE('',(#777),#468,.T.);
#3974=ADVANCED_FACE('',(#778),#511,.T.);
#3975=ADVANCED_FACE('',(#779),#469,.T.);
#3976=ADVANCED_FACE('',(#780),#470,.T.);
#3977=ADVANCED_FACE('',(#781),#3817,.T.);
#3978=ADVANCED_FACE('',(#782),#471,.T.);
#3979=ADVANCED_FACE('',(#783),#3818,.T.);
#3980=ADVANCED_FACE('',(#784),#3819,.T.);
#3981=ADVANCED_FACE('',(#785),#472,.T.);
#3982=ADVANCED_FACE('',(#786),#3820,.T.);
#3983=ADVANCED_FACE('',(#787),#473,.F.);
#3984=ADVANCED_FACE('',(#788),#512,.T.);
#3985=ADVANCED_FACE('',(#789),#474,.T.);
#3986=ADVANCED_FACE('',(#790),#513,.T.);
#3987=ADVANCED_FACE('',(#791),#475,.T.);
#3988=ADVANCED_FACE('',(#792),#514,.T.);
#3989=ADVANCED_FACE('',(#793),#476,.T.);
#3990=ADVANCED_FACE('',(#794),#515,.T.);
#3991=ADVANCED_FACE('',(#795),#477,.T.);
#3992=ADVANCED_FACE('',(#796),#516,.T.);
#3993=ADVANCED_FACE('',(#797),#478,.T.);
#3994=ADVANCED_FACE('',(#798),#517,.T.);
#3995=ADVANCED_FACE('',(#799),#479,.T.);
#3996=ADVANCED_FACE('',(#800),#518,.T.);
#3997=ADVANCED_FACE('',(#801),#480,.T.);
#3998=ADVANCED_FACE('',(#802),#3821,.T.);
#3999=ADVANCED_FACE('',(#803),#481,.F.);
#4000=ADVANCED_FACE('',(#804),#3822,.T.);
#4001=ADVANCED_FACE('',(#805),#482,.T.);
#4002=ADVANCED_FACE('',(#806),#3823,.T.);
#4003=ADVANCED_FACE('',(#807),#483,.T.);
#4004=ADVANCED_FACE('',(#808,#392),#3824,.T.);
#4005=ADVANCED_FACE('',(#809,#393),#3825,.T.);
#4039=CLOSED_SHELL('',(#3953,#3954,#3955,#3956,#3957,#3958,#3959,#3960,
#3961,#3962,#3963,#3964,#3965,#3966,#3967,#3968,#3969,#3970,#3971,#3972,
#3973,#3974,#3975,#3976,#3977,#3978,#3979,#3980,#3981,#3982,#3983,#3984,
#3985,#3986,#3987,#3988,#3989,#3990,#3991,#3992,#3993,#3994,#3995,#3996,
#3997,#3998,#3999,#4000,#4001,#4002,#4003,#4004,#4005));
#4317=AXIS2_PLACEMENT_3D('',#33620,#4954,#4955);
#4318=AXIS2_PLACEMENT_3D('',#33621,#4956,#4957);
#4319=AXIS2_PLACEMENT_3D('',#33733,#4959,#4960);
#4320=AXIS2_PLACEMENT_3D('',#33876,#4961,#4962);
#4321=AXIS2_PLACEMENT_3D('',#34057,#4964,#4965);
#4322=AXIS2_PLACEMENT_3D('',#34269,#4966,#4967);
#4323=AXIS2_PLACEMENT_3D('',#34280,#4969,#4970);
#4324=AXIS2_PLACEMENT_3D('',#34410,#4971,#4972);
#4325=AXIS2_PLACEMENT_3D('',#34712,#4974,#4975);
#4326=AXIS2_PLACEMENT_3D('',#34717,#4977,#4978);
#4327=AXIS2_PLACEMENT_3D('',#35730,#4979,#4980);
#4328=AXIS2_PLACEMENT_3D('',#35955,#4981,#4982);
#4329=AXIS2_PLACEMENT_3D('',#35956,#4983,#4984);
#4330=AXIS2_PLACEMENT_3D('',#36719,#4985,#4986);
#4331=AXIS2_PLACEMENT_3D('',#36722,#4987,#4988);
#4332=AXIS2_PLACEMENT_3D('',#36724,#4989,#4990);
#4333=AXIS2_PLACEMENT_3D('',#36726,#4991,#4992);
#4334=AXIS2_PLACEMENT_3D('',#36727,#4993,#4994);
#4335=AXIS2_PLACEMENT_3D('',#36728,#4995,#4996);
#4336=AXIS2_PLACEMENT_3D('',#36731,#4997,#4998);
#4337=AXIS2_PLACEMENT_3D('',#36734,#5001,#5002);
#4338=AXIS2_PLACEMENT_3D('',#36737,#5003,#5004);
#4339=AXIS2_PLACEMENT_3D('',#36738,#5005,#5006);
#4340=AXIS2_PLACEMENT_3D('',#36739,#5007,#5008);
#4341=AXIS2_PLACEMENT_3D('',#36740,#5009,#5010);
#4342=AXIS2_PLACEMENT_3D('',#36743,#5011,#5012);
#4343=AXIS2_PLACEMENT_3D('',#36746,#5015,#5016);
#4344=AXIS2_PLACEMENT_3D('',#36749,#5017,#5018);
#4345=AXIS2_PLACEMENT_3D('',#36750,#5019,#5020);
#4346=AXIS2_PLACEMENT_3D('',#36751,#5021,#5022);
#4347=AXIS2_PLACEMENT_3D('',#36752,#5023,#5024);
#4348=AXIS2_PLACEMENT_3D('',#36755,#5025,#5026);
#4349=AXIS2_PLACEMENT_3D('',#36758,#5029,#5030);
#4350=AXIS2_PLACEMENT_3D('',#36761,#5031,#5032);
#4351=AXIS2_PLACEMENT_3D('',#36762,#5033,#5034);
#4352=AXIS2_PLACEMENT_3D('',#36763,#5035,#5036);
#4353=AXIS2_PLACEMENT_3D('',#36764,#5037,#5038);
#4354=AXIS2_PLACEMENT_3D('',#36767,#5039,#5040);
#4355=AXIS2_PLACEMENT_3D('',#36770,#5043,#5044);
#4356=AXIS2_PLACEMENT_3D('',#36773,#5045,#5046);
#4357=AXIS2_PLACEMENT_3D('',#36774,#5047,#5048);
#4358=AXIS2_PLACEMENT_3D('',#36775,#5049,#5050);
#4359=AXIS2_PLACEMENT_3D('',#36776,#5051,#5052);
#4360=AXIS2_PLACEMENT_3D('',#36779,#5053,#5054);
#4361=AXIS2_PLACEMENT_3D('',#36782,#5057,#5058);
#4362=AXIS2_PLACEMENT_3D('',#36785,#5059,#5060);
#4363=AXIS2_PLACEMENT_3D('',#36786,#5061,#5062);
#4364=AXIS2_PLACEMENT_3D('',#36787,#5063,#5064);
#4365=AXIS2_PLACEMENT_3D('',#36788,#5065,#5066);
#4366=AXIS2_PLACEMENT_3D('',#36791,#5067,#5068);
#4367=AXIS2_PLACEMENT_3D('',#36794,#5071,#5072);
#4368=AXIS2_PLACEMENT_3D('',#36797,#5073,#5074);
#4369=AXIS2_PLACEMENT_3D('',#36798,#5075,#5076);
#4370=AXIS2_PLACEMENT_3D('',#36799,#5077,#5078);
#4371=AXIS2_PLACEMENT_3D('',#36800,#5079,#5080);
#4372=AXIS2_PLACEMENT_3D('',#36803,#5083,#5084);
#4373=AXIS2_PLACEMENT_3D('',#36807,#5086,#5087);
#4374=AXIS2_PLACEMENT_3D('',#36809,#5089,#5090);
#4375=AXIS2_PLACEMENT_3D('',#36813,#5093,#5094);
#4376=AXIS2_PLACEMENT_3D('',#36816,#5096,#5097);
#4377=AXIS2_PLACEMENT_3D('',#36817,#5098,#5099);
#4378=AXIS2_PLACEMENT_3D('',#36823,#5102,#5103);
#4379=AXIS2_PLACEMENT_3D('',#36827,#5105,#5106);
#4380=AXIS2_PLACEMENT_3D('',#36829,#5108,#5109);
#4381=AXIS2_PLACEMENT_3D('',#36831,#5111,#5112);
#4382=AXIS2_PLACEMENT_3D('',#36834,#5115,#5116);
#4383=AXIS2_PLACEMENT_3D('',#36836,#5118,#5119);
#4384=AXIS2_PLACEMENT_3D('',#36837,#5120,#5121);
#4385=AXIS2_PLACEMENT_3D('',#36840,#5122,#5123);
#4386=AXIS2_PLACEMENT_3D('',#36842,#5124,#5125);
#4387=AXIS2_PLACEMENT_3D('',#36844,#5126,#5127);
#4388=AXIS2_PLACEMENT_3D('',#36845,#5128,#5129);
#4389=AXIS2_PLACEMENT_3D('',#36846,#5130,#5131);
#4390=AXIS2_PLACEMENT_3D('',#36849,#5132,#5133);
#4391=AXIS2_PLACEMENT_3D('',#36852,#5136,#5137);
#4392=AXIS2_PLACEMENT_3D('',#36855,#5138,#5139);
#4393=AXIS2_PLACEMENT_3D('',#36856,#5140,#5141);
#4394=AXIS2_PLACEMENT_3D('',#36857,#5142,#5143);
#4395=AXIS2_PLACEMENT_3D('',#36858,#5144,#5145);
#4396=AXIS2_PLACEMENT_3D('',#36860,#5146,#5147);
#4397=AXIS2_PLACEMENT_3D('',#36863,#5150,#5151);
#4398=AXIS2_PLACEMENT_3D('',#36865,#5152,#5153);
#4399=AXIS2_PLACEMENT_3D('',#36866,#5154,#5155);
#4400=AXIS2_PLACEMENT_3D('',#36867,#5156,#5157);
#4401=AXIS2_PLACEMENT_3D('',#36869,#5158,#5159);
#4402=AXIS2_PLACEMENT_3D('',#36871,#5161,#5162);
#4403=AXIS2_PLACEMENT_3D('',#36873,#5163,#5164);
#4404=AXIS2_PLACEMENT_3D('',#36874,#5165,#5166);
#4405=AXIS2_PLACEMENT_3D('',#36875,#5167,#5168);
#4406=AXIS2_PLACEMENT_3D('',#36877,#5169,#5170);
#4407=AXIS2_PLACEMENT_3D('',#36879,#5172,#5173);
#4408=AXIS2_PLACEMENT_3D('',#36881,#5174,#5175);
#4409=AXIS2_PLACEMENT_3D('',#36882,#5176,#5177);
#4410=AXIS2_PLACEMENT_3D('',#36883,#5178,#5179);
#4411=AXIS2_PLACEMENT_3D('',#36885,#5180,#5181);
#4412=AXIS2_PLACEMENT_3D('',#36887,#5183,#5184);
#4413=AXIS2_PLACEMENT_3D('',#36889,#5185,#5186);
#4414=AXIS2_PLACEMENT_3D('',#36890,#5187,#5188);
#4415=AXIS2_PLACEMENT_3D('',#36891,#5189,#5190);
#4416=AXIS2_PLACEMENT_3D('',#36893,#5191,#5192);
#4417=AXIS2_PLACEMENT_3D('',#36895,#5194,#5195);
#4418=AXIS2_PLACEMENT_3D('',#36898,#5196,#5197);
#4419=AXIS2_PLACEMENT_3D('',#36899,#5198,#5199);
#4420=AXIS2_PLACEMENT_3D('',#36900,#5200,#5201);
#4421=AXIS2_PLACEMENT_3D('',#36901,#5202,#5203);
#4422=AXIS2_PLACEMENT_3D('',#36904,#5206,#5207);
#4423=AXIS2_PLACEMENT_3D('',#36906,#5209,#5210);
#4424=AXIS2_PLACEMENT_3D('',#36909,#5213,#5214);
#4425=AXIS2_PLACEMENT_3D('',#36911,#5216,#5217);
#4426=AXIS2_PLACEMENT_3D('',#36912,#5218,#5219);
#4427=AXIS2_PLACEMENT_3D('',#36914,#5221,#5222);
#4428=AXIS2_PLACEMENT_3D('',#36915,#5223,#5224);
#4429=AXIS2_PLACEMENT_3D('',#36916,#5225,#5226);
#4954=DIRECTION('axis',(0.,0.,1.));
#4955=DIRECTION('refdir',(1.,0.,0.));
#4956=DIRECTION('center_axis',(0.,0.,1.));
#4957=DIRECTION('ref_axis',(-1.,0.,0.));
#4958=DIRECTION('',(0.,0.,1.));
#4959=DIRECTION('center_axis',(0.,0.,-1.));
#4960=DIRECTION('ref_axis',(-1.,0.,0.));
#4961=DIRECTION('center_axis',(0.,0.,1.));
#4962=DIRECTION('ref_axis',(-1.,0.,0.));
#4963=DIRECTION('',(0.,0.,1.));
#4964=DIRECTION('center_axis',(0.,0.,1.));
#4965=DIRECTION('ref_axis',(-1.,0.,0.));
#4966=DIRECTION('center_axis',(0.,0.,1.));
#4967=DIRECTION('ref_axis',(0.457762905907022,0.889074306217179,0.));
#4968=DIRECTION('',(0.,0.,1.));
#4969=DIRECTION('center_axis',(0.,0.,-1.));
#4970=DIRECTION('ref_axis',(0.457762905907022,0.889074306217179,0.));
#4971=DIRECTION('center_axis',(0.,0.,1.));
#4972=DIRECTION('ref_axis',(0.457762905907022,0.889074306217179,0.));
#4973=DIRECTION('',(0.,0.,1.));
#4974=DIRECTION('center_axis',(0.,0.,1.));
#4975=DIRECTION('ref_axis',(0.457762905907022,0.889074306217179,0.));
#4976=DIRECTION('',(0.,0.,1.));
#4977=DIRECTION('center_axis',(0.,0.,1.));
#4978=DIRECTION('ref_axis',(0.457762905907022,0.889074306217179,0.));
#4979=DIRECTION('center_axis',(0.,0.,1.));
#4980=DIRECTION('ref_axis',(0.457762905907022,0.889074306217179,0.));
#4981=DIRECTION('center_axis',(0.,0.,1.));
#4982=DIRECTION('ref_axis',(0.457762905907022,0.889074306217179,0.));
#4983=DIRECTION('center_axis',(0.,0.,1.));
#4984=DIRECTION('ref_axis',(-1.,0.,0.));
#4985=DIRECTION('center_axis',(-1.,0.,0.));
#4986=DIRECTION('ref_axis',(0.,0.,1.));
#4987=DIRECTION('center_axis',(0.,1.,0.));
#4988=DIRECTION('ref_axis',(0.,0.,-1.));
#4989=DIRECTION('center_axis',(-1.,0.,0.));
#4990=DIRECTION('ref_axis',(0.,0.382683432365091,0.923879532511286));
#4991=DIRECTION('center_axis',(0.,-0.707106781186548,0.707106781186548));
#4992=DIRECTION('ref_axis',(-1.,0.,0.));
#4993=DIRECTION('center_axis',(1.,0.,0.));
#4994=DIRECTION('ref_axis',(0.,0.382683432365091,0.923879532511286));
#4995=DIRECTION('center_axis',(0.,-0.707106781186547,0.707106781186548));
#4996=DIRECTION('ref_axis',(-0.707106781186549,-0.499999999999999,-0.499999999999999));
#4997=DIRECTION('center_axis',(0.,-0.707106781186554,0.707106781186541));
#4998=DIRECTION('ref_axis',(-1.,0.,0.));
#4999=DIRECTION('',(0.,-0.707106781186547,0.707106781186548));
#5000=DIRECTION('',(0.,0.707106781186547,-0.707106781186548));
#5001=DIRECTION('center_axis',(1.,0.,0.));
#5002=DIRECTION('ref_axis',(0.,0.,-1.));
#5003=DIRECTION('center_axis',(0.,-1.,0.));
#5004=DIRECTION('ref_axis',(-1.,0.,0.));
#5005=DIRECTION('center_axis',(-1.,0.,0.));
#5006=DIRECTION('ref_axis',(0.,-0.38268343236509,-0.923879532511287));
#5007=DIRECTION('center_axis',(1.,0.,0.));
#5008=DIRECTION('ref_axis',(0.,-0.38268343236509,-0.923879532511287));
#5009=DIRECTION('center_axis',(0.,-1.,0.));
#5010=DIRECTION('ref_axis',(-0.707106781186549,0.,-0.707106781186546));
#5011=DIRECTION('center_axis',(0.,-1.,0.));
#5012=DIRECTION('ref_axis',(-1.,0.,0.));
#5013=DIRECTION('',(0.,-1.,0.));
#5014=DIRECTION('',(0.,1.,0.));
#5015=DIRECTION('center_axis',(0.,0.,1.));
#5016=DIRECTION('ref_axis',(1.,0.,0.));
#5017=DIRECTION('center_axis',(-1.,0.,0.));
#5018=DIRECTION('ref_axis',(0.,1.,0.));
#5019=DIRECTION('center_axis',(0.,0.,1.));
#5020=DIRECTION('ref_axis',(-0.707106781186547,0.707106781186547,0.));
#5021=DIRECTION('center_axis',(0.,0.,-1.));
#5022=DIRECTION('ref_axis',(-0.707106781186548,0.707106781186548,0.));
#5023=DIRECTION('center_axis',(1.,0.,0.));
#5024=DIRECTION('ref_axis',(0.,0.707106781186549,-0.707106781186546));
#5025=DIRECTION('center_axis',(-1.,0.,0.));
#5026=DIRECTION('ref_axis',(0.,1.,0.));
#5027=DIRECTION('',(-1.,0.,0.));
#5028=DIRECTION('',(1.,0.,0.));
#5029=DIRECTION('center_axis',(0.,0.,1.));
#5030=DIRECTION('ref_axis',(1.,0.,0.));
#5031=DIRECTION('center_axis',(0.,1.,0.));
#5032=DIRECTION('ref_axis',(1.,0.,0.));
#5033=DIRECTION('center_axis',(0.,0.,1.));
#5034=DIRECTION('ref_axis',(0.707106781186547,0.707106781186547,0.));
#5035=DIRECTION('center_axis',(0.,0.,-1.));
#5036=DIRECTION('ref_axis',(0.707106781186548,0.707106781186548,0.));
#5037=DIRECTION('center_axis',(0.,1.,0.));
#5038=DIRECTION('ref_axis',(0.707106781186549,0.,-0.707106781186546));
#5039=DIRECTION('center_axis',(0.,1.,-2.22044604925032E-15));
#5040=DIRECTION('ref_axis',(1.,0.,0.));
#5041=DIRECTION('',(0.,1.,0.));
#5042=DIRECTION('',(0.,-1.,0.));
#5043=DIRECTION('center_axis',(-1.,0.,0.));
#5044=DIRECTION('ref_axis',(0.,0.,1.));
#5045=DIRECTION('center_axis',(0.,0.707106781186548,-0.707106781186548));
#5046=DIRECTION('ref_axis',(1.,0.,0.));
#5047=DIRECTION('center_axis',(1.,0.,0.));
#5048=DIRECTION('ref_axis',(0.,-0.38268343236509,-0.923879532511287));
#5049=DIRECTION('center_axis',(-1.,0.,0.));
#5050=DIRECTION('ref_axis',(0.,-0.38268343236509,-0.923879532511287));
#5051=DIRECTION('center_axis',(0.,0.707106781186547,-0.707106781186548));
#5052=DIRECTION('ref_axis',(0.707106781186549,-0.499999999999999,-0.499999999999999));
#5053=DIRECTION('center_axis',(0.,0.707106781186552,-0.707106781186543));
#5054=DIRECTION('ref_axis',(1.,0.,0.));
#5055=DIRECTION('',(0.,0.707106781186547,-0.707106781186548));
#5056=DIRECTION('',(0.,-0.707106781186547,0.707106781186548));
#5057=DIRECTION('center_axis',(1.,0.,0.));
#5058=DIRECTION('ref_axis',(0.,0.,-1.));
#5059=DIRECTION('center_axis',(0.,1.,0.));
#5060=DIRECTION('ref_axis',(1.,0.,0.));
#5061=DIRECTION('center_axis',(-1.,0.,0.));
#5062=DIRECTION('ref_axis',(0.,0.382683432365091,0.923879532511286));
#5063=DIRECTION('center_axis',(1.,0.,0.));
#5064=DIRECTION('ref_axis',(0.,0.382683432365091,0.923879532511286));
#5065=DIRECTION('center_axis',(0.,1.,0.));
#5066=DIRECTION('ref_axis',(0.707106781186555,0.,-0.70710678118654));
#5067=DIRECTION('center_axis',(0.,1.,0.));
#5068=DIRECTION('ref_axis',(1.,0.,0.));
#5069=DIRECTION('',(0.,1.,0.));
#5070=DIRECTION('',(0.,-1.,0.));
#5071=DIRECTION('center_axis',(0.,0.,1.));
#5072=DIRECTION('ref_axis',(1.,0.,0.));
#5073=DIRECTION('center_axis',(0.,-1.,0.));
#5074=DIRECTION('ref_axis',(-1.,0.,0.));
#5075=DIRECTION('center_axis',(0.,0.,1.));
#5076=DIRECTION('ref_axis',(0.,-1.,0.));
#5077=DIRECTION('center_axis',(0.,0.,-1.));
#5078=DIRECTION('ref_axis',(0.,-1.,0.));
#5079=DIRECTION('center_axis',(0.,-1.,0.));
#5080=DIRECTION('ref_axis',(-0.707106781186555,0.,-0.70710678118654));
#5081=DIRECTION('',(0.,1.,0.));
#5082=DIRECTION('',(0.,-1.,0.));
#5083=DIRECTION('center_axis',(0.,0.,1.));
#5084=DIRECTION('ref_axis',(0.707106781186548,0.707106781186548,0.));
#5085=DIRECTION('',(0.,0.,1.));
#5086=DIRECTION('center_axis',(0.,0.,1.));
#5087=DIRECTION('ref_axis',(0.707106781186548,0.707106781186548,0.));
#5088=DIRECTION('',(0.,0.,-1.));
#5089=DIRECTION('center_axis',(0.,1.,0.));
#5090=DIRECTION('ref_axis',(0.,0.,1.));
#5091=DIRECTION('',(0.,0.,-1.));
#5092=DIRECTION('',(-1.,0.,0.));
#5093=DIRECTION('center_axis',(0.,0.,-1.));
#5094=DIRECTION('ref_axis',(-0.707106781186548,0.707106781186548,0.));
#5095=DIRECTION('',(0.,0.,1.));
#5096=DIRECTION('center_axis',(0.,0.,1.));
#5097=DIRECTION('ref_axis',(-0.707106781186548,0.707106781186548,0.));
#5098=DIRECTION('center_axis',(-1.,0.,0.));
#5099=DIRECTION('ref_axis',(0.,0.,1.));
#5100=DIRECTION('',(0.,0.,-1.));
#5101=DIRECTION('',(0.,-1.,0.));
#5102=DIRECTION('center_axis',(1.,0.,0.));
#5103=DIRECTION('ref_axis',(0.,0.382683432365091,0.923879532511286));
#5104=DIRECTION('',(0.,-0.707106781186547,0.707106781186548));
#5105=DIRECTION('center_axis',(-1.,0.,0.));
#5106=DIRECTION('ref_axis',(0.,-0.38268343236509,-0.923879532511287));
#5107=DIRECTION('',(0.,-1.,0.));
#5108=DIRECTION('center_axis',(0.,0.,-1.));
#5109=DIRECTION('ref_axis',(0.,1.,0.));
#5110=DIRECTION('',(-1.,0.,0.));
#5111=DIRECTION('center_axis',(1.,0.,0.));
#5112=DIRECTION('ref_axis',(0.,-0.38268343236509,-0.923879532511287));
#5113=DIRECTION('',(-1.,0.,0.));
#5114=DIRECTION('',(1.,0.,0.));
#5115=DIRECTION('center_axis',(0.,-0.707106781186548,-0.707106781186547));
#5116=DIRECTION('ref_axis',(0.,0.707106781186547,-0.707106781186548));
#5117=DIRECTION('',(1.,0.,0.));
#5118=DIRECTION('center_axis',(1.,0.,0.));
#5119=DIRECTION('ref_axis',(0.,0.38268343236509,0.923879532511287));
#5120=DIRECTION('center_axis',(-1.,0.,0.));
#5121=DIRECTION('ref_axis',(0.,0.,1.));
#5122=DIRECTION('center_axis',(0.,1.,0.));
#5123=DIRECTION('ref_axis',(0.,0.,1.));
#5124=DIRECTION('center_axis',(-1.,0.,0.));
#5125=DIRECTION('ref_axis',(0.,0.382683432365091,0.923879532511286));
#5126=DIRECTION('center_axis',(0.,-0.707106781186539,0.707106781186556));
#5127=DIRECTION('ref_axis',(1.,0.,0.));
#5128=DIRECTION('center_axis',(1.,0.,0.));
#5129=DIRECTION('ref_axis',(0.,0.382683432365091,0.923879532511286));
#5130=DIRECTION('center_axis',(0.,-0.707106781186547,0.707106781186548));
#5131=DIRECTION('ref_axis',(0.707106781186549,0.499999999999999,0.499999999999999));
#5132=DIRECTION('center_axis',(0.,-0.707106781186545,0.70710678118655));
#5133=DIRECTION('ref_axis',(1.,0.,0.));
#5134=DIRECTION('',(0.,-0.707106781186547,0.707106781186548));
#5135=DIRECTION('',(0.,0.707106781186547,-0.707106781186548));
#5136=DIRECTION('center_axis',(1.,0.,0.));
#5137=DIRECTION('ref_axis',(0.,0.,-1.));
#5138=DIRECTION('center_axis',(0.,-1.,0.));
#5139=DIRECTION('ref_axis',(1.,0.,0.));
#5140=DIRECTION('center_axis',(-1.,0.,0.));
#5141=DIRECTION('ref_axis',(0.,-0.38268343236509,-0.923879532511287));
#5142=DIRECTION('center_axis',(1.,0.,0.));
#5143=DIRECTION('ref_axis',(0.,-0.38268343236509,-0.923879532511287));
#5144=DIRECTION('center_axis',(0.,-1.,0.));
#5145=DIRECTION('ref_axis',(0.707106781186549,0.,0.707106781186546));
#5146=DIRECTION('center_axis',(0.,-1.,0.));
#5147=DIRECTION('ref_axis',(1.,0.,0.));
#5148=DIRECTION('',(0.,-1.,0.));
#5149=DIRECTION('',(0.,1.,0.));
#5150=DIRECTION('center_axis',(0.,0.,-1.));
#5151=DIRECTION('ref_axis',(-1.,0.,0.));
#5152=DIRECTION('center_axis',(1.,0.,0.));
#5153=DIRECTION('ref_axis',(0.,1.,0.));
#5154=DIRECTION('center_axis',(0.,0.,-1.));
#5155=DIRECTION('ref_axis',(0.707106781186547,0.707106781186547,0.));
#5156=DIRECTION('center_axis',(1.,0.,0.));
#5157=DIRECTION('ref_axis',(0.,0.707106781186549,0.707106781186546));
#5158=DIRECTION('center_axis',(1.,0.,0.));
#5159=DIRECTION('ref_axis',(0.,1.,0.));
#5160=DIRECTION('',(1.,0.,0.));
#5161=DIRECTION('center_axis',(0.,0.,-1.));
#5162=DIRECTION('ref_axis',(-1.,0.,0.));
#5163=DIRECTION('center_axis',(0.,1.,0.));
#5164=DIRECTION('ref_axis',(-1.,0.,0.));
#5165=DIRECTION('center_axis',(0.,0.,-1.));
#5166=DIRECTION('ref_axis',(-0.707106781186547,0.707106781186547,0.));
#5167=DIRECTION('center_axis',(0.,1.,0.));
#5168=DIRECTION('ref_axis',(-0.707106781186549,0.,0.707106781186546));
#5169=DIRECTION('center_axis',(0.,1.,0.));
#5170=DIRECTION('ref_axis',(-1.,0.,0.));
#5171=DIRECTION('',(0.,1.,0.));
#5172=DIRECTION('center_axis',(-1.,0.,0.));
#5173=DIRECTION('ref_axis',(0.,0.,1.));
#5174=DIRECTION('center_axis',(0.,0.707106781186545,-0.70710678118655));
#5175=DIRECTION('ref_axis',(-1.,0.,0.));
#5176=DIRECTION('center_axis',(1.,0.,0.));
#5177=DIRECTION('ref_axis',(0.,-0.38268343236509,-0.923879532511287));
#5178=DIRECTION('center_axis',(0.,0.707106781186547,-0.707106781186548));
#5179=DIRECTION('ref_axis',(-0.707106781186549,0.499999999999999,0.499999999999999));
#5180=DIRECTION('center_axis',(0.,0.707106781186548,-0.707106781186548));
#5181=DIRECTION('ref_axis',(-1.,0.,0.));
#5182=DIRECTION('',(0.,0.707106781186547,-0.707106781186548));
#5183=DIRECTION('center_axis',(1.,0.,0.));
#5184=DIRECTION('ref_axis',(0.,0.,-1.));
#5185=DIRECTION('center_axis',(0.,1.,0.));
#5186=DIRECTION('ref_axis',(-1.,0.,0.));
#5187=DIRECTION('center_axis',(-1.,0.,0.));
#5188=DIRECTION('ref_axis',(0.,0.382683432365091,0.923879532511286));
#5189=DIRECTION('center_axis',(0.,1.,0.));
#5190=DIRECTION('ref_axis',(-0.707106781186543,0.,0.707106781186552));
#5191=DIRECTION('center_axis',(0.,1.,0.));
#5192=DIRECTION('ref_axis',(-1.,0.,0.));
#5193=DIRECTION('',(0.,1.,0.));
#5194=DIRECTION('center_axis',(0.,0.,-1.));
#5195=DIRECTION('ref_axis',(-1.,0.,0.));
#5196=DIRECTION('center_axis',(0.,-1.,0.));
#5197=DIRECTION('ref_axis',(1.,0.,0.));
#5198=DIRECTION('center_axis',(0.,0.,-1.));
#5199=DIRECTION('ref_axis',(0.,-1.,0.));
#5200=DIRECTION('center_axis',(0.,0.,1.));
#5201=DIRECTION('ref_axis',(0.,-1.,0.));
#5202=DIRECTION('center_axis',(0.,-1.,0.));
#5203=DIRECTION('ref_axis',(0.707106781186543,0.,0.707106781186552));
#5204=DIRECTION('',(0.,1.,0.));
#5205=DIRECTION('',(0.,-1.,0.));
#5206=DIRECTION('center_axis',(0.,0.,1.));
#5207=DIRECTION('ref_axis',(0.,-1.,0.));
#5208=DIRECTION('',(1.,0.,0.));
#5209=DIRECTION('center_axis',(-1.,0.,0.));
#5210=DIRECTION('ref_axis',(0.,-0.38268343236509,-0.923879532511287));
#5211=DIRECTION('',(1.,0.,0.));
#5212=DIRECTION('',(-1.,0.,0.));
#5213=DIRECTION('center_axis',(0.,0.707106781186548,0.707106781186547));
#5214=DIRECTION('ref_axis',(0.,-0.707106781186547,0.707106781186548));
#5215=DIRECTION('',(-1.,0.,0.));
#5216=DIRECTION('center_axis',(1.,0.,0.));
#5217=DIRECTION('ref_axis',(0.,0.38268343236509,0.923879532511287));
#5218=DIRECTION('center_axis',(1.,0.,0.));
#5219=DIRECTION('ref_axis',(0.,0.,-1.));
#5220=DIRECTION('',(0.,0.,1.));
#5221=DIRECTION('center_axis',(0.,0.,1.));
#5222=DIRECTION('ref_axis',(-0.707106781186548,-0.707106781186548,0.));
#5223=DIRECTION('center_axis',(0.,0.,-1.));
#5224=DIRECTION('ref_axis',(0.,1.,0.));
#5225=DIRECTION('center_axis',(0.,0.,1.));
#5226=DIRECTION('ref_axis',(0.,-1.,0.));
#33620=CARTESIAN_POINT('',(0.,0.,0.));
#33621=CARTESIAN_POINT('Origin',(0.,0.,32.));
#33622=CARTESIAN_POINT('',(3.93496388660084,0.00195648875352047,37.2208358380349));
#33623=CARTESIAN_POINT('',(3.93463686453598,0.00228919349351085,37.4041629160656));
#33624=CARTESIAN_POINT('',(3.933,4.81653586104654E-16,32.));
#33625=CARTESIAN_POINT('',(-3.88542223618671,0.609904128979188,37.9980892280756));
#33626=CARTESIAN_POINT('Ctrl Pts',(-3.88542223618671,0.609904128979188,
37.9980892280756));
#33627=CARTESIAN_POINT('Ctrl Pts',(-3.86749256473595,0.724125923573192,
37.9922268209659));
#33628=CARTESIAN_POINT('Ctrl Pts',(-3.84449896610055,0.837702284267991,
37.9863644138562));
#33629=CARTESIAN_POINT('Ctrl Pts',(-3.81650392804124,0.950150918141841,
37.9805020067465));
#33630=CARTESIAN_POINT('Ctrl Pts',(-3.78853529915897,1.06249347336439,37.9746451299506));
#33631=CARTESIAN_POINT('Ctrl Pts',(-3.75557471545758,1.17371001885672,37.9687882531547));
#33632=CARTESIAN_POINT('Ctrl Pts',(-3.71773598028384,1.28332699687297,37.9629313763589));
#33633=CARTESIAN_POINT('Ctrl Pts',(-3.67990854063047,1.39291125231526,37.9570762479426));
#33634=CARTESIAN_POINT('Ctrl Pts',(-3.6372059613303,1.5008964937652,37.9512211195263));
#33635=CARTESIAN_POINT('Ctrl Pts',(-3.58979229255919,1.60682304448332,37.94536599111));
#33636=CARTESIAN_POINT('Ctrl Pts',(-3.54240969388923,1.71268018170253,37.93951469955));
#33637=CARTESIAN_POINT('Ctrl Pts',(-3.49032233155603,1.81648094151968,37.9336634079899));
#33638=CARTESIAN_POINT('Ctrl Pts',(-3.43374231814287,1.91778588288548,37.9278121164299));
#33639=CARTESIAN_POINT('Ctrl Pts',(-3.37716709289371,2.01908225117672,37.9219613200437));
#33640=CARTESIAN_POINT('Ctrl Pts',(-3.31610017418119,2.11788286012534,37.9161105236576));
#33641=CARTESIAN_POINT('Ctrl Pts',(-3.25079938729001,2.21377332705832,37.9102597272714));
#33642=CARTESIAN_POINT('Ctrl Pts',(-3.18548831005988,2.3096789047649,37.9044080088952));
#33643=CARTESIAN_POINT('Ctrl Pts',(-3.11594227087696,2.40267308700958,37.8985562905189));
#33644=CARTESIAN_POINT('Ctrl Pts',(-3.04246171385679,2.4923715051564,37.8927045721426));
#33645=CARTESIAN_POINT('Ctrl Pts',(-2.9689019872486,2.58216656637588,37.8868465489947));
#33646=CARTESIAN_POINT('Ctrl Pts',(-2.89139953671942,2.66865844926548,37.8809885258468));
#33647=CARTESIAN_POINT('Ctrl Pts',(-2.81029448477806,2.75149666705704,37.8751305026989));
#33648=CARTESIAN_POINT('Ctrl Pts',(-2.72914963764217,2.83437553044236,37.8692696052397));
#33649=CARTESIAN_POINT('Ctrl Pts',(-2.6443989705447,2.91359687583261,37.8634087077804));
#33650=CARTESIAN_POINT('Ctrl Pts',(-2.55641735766959,2.98884915869062,37.8575478103212));
#33651=CARTESIAN_POINT('Ctrl Pts',(-2.46828756305929,3.06422818409729,37.8516770417317));
#33652=CARTESIAN_POINT('Ctrl Pts',(-2.37691627453245,3.13562453343064,37.8458062731423));
#33653=CARTESIAN_POINT('Ctrl Pts',(-2.28270965334754,3.20276843348281,37.8399355045529));
#33654=CARTESIAN_POINT('Ctrl Pts',(-2.18895820069543,3.26958792119445,37.8340931011578));
#33655=CARTESIAN_POINT('Ctrl Pts',(-2.0923991372675,3.33219581956083,37.8282506977628));
#33656=CARTESIAN_POINT('Ctrl Pts',(-1.99345630322199,3.39037180367353,37.8224082943678));
#33657=CARTESIAN_POINT('Ctrl Pts',(-1.89401014270797,3.44884373152909,37.8165361704145));
#33658=CARTESIAN_POINT('Ctrl Pts',(-1.79182243863938,3.5030345546936,37.8106640464611));
#33659=CARTESIAN_POINT('Ctrl Pts',(-1.68729798416966,3.55267709095789,37.8047919225078));
#33660=CARTESIAN_POINT('Ctrl Pts',(-1.58290904772492,3.60225526469091,37.7989274118794));
#33661=CARTESIAN_POINT('Ctrl Pts',(-1.47618975572388,3.64729670268684,37.7930629012511));
#33662=CARTESIAN_POINT('Ctrl Pts',(-1.36757205913616,3.68757856364716,37.7871983906227));
#33663=CARTESIAN_POINT('Ctrl Pts',(-1.25906612907142,3.72781897497561,37.7813399145171));
#33664=CARTESIAN_POINT('Ctrl Pts',(-1.14866606518523,3.76330940785714,37.7754814384116));
#33665=CARTESIAN_POINT('Ctrl Pts',(-1.03682588890287,3.79387415132616,37.769622962306));
#33666=CARTESIAN_POINT('Ctrl Pts',(-0.920575705995505,3.82564410320659,
37.7635334787101));
#33667=CARTESIAN_POINT('Ctrl Pts',(-0.802769914156219,3.85209172586888,
37.7574439951142));
#33668=CARTESIAN_POINT('Ctrl Pts',(-0.683938671629199,3.87307589564807,
37.7513545115183));
#33669=CARTESIAN_POINT('Ctrl Pts',(-0.569747881856857,3.89324061722167,
37.7455028270089));
#33670=CARTESIAN_POINT('Ctrl Pts',(-0.454610673238864,3.90836050408855,
37.7396511424996));
#33671=CARTESIAN_POINT('Ctrl Pts',(-0.339009367189833,3.91836211304641,
37.7337994579902));
#33672=CARTESIAN_POINT('Ctrl Pts',(-0.223425692845461,3.92836219654214,
37.7279486659896));
#33673=CARTESIAN_POINT('Ctrl Pts',(-0.107378473573039,3.93324551867752,
37.722097873989));
#33674=CARTESIAN_POINT('Ctrl Pts',(0.00864472130136986,3.93299049945377,
37.7162470819884));
#33675=CARTESIAN_POINT('Ctrl Pts',(0.124678322130959,3.93273545735771,37.7103957652385));
#33676=CARTESIAN_POINT('Ctrl Pts',(0.240687480842907,3.92734115868281,37.7045444484887));
#33677=CARTESIAN_POINT('Ctrl Pts',(0.356185216416442,3.91683814978439,37.6986931317389));
#33678=CARTESIAN_POINT('Ctrl Pts',(0.471721285545492,3.90633165495031,37.6928398729442));
#33679=CARTESIAN_POINT('Ctrl Pts',(0.586745182521605,3.89071311577341,37.6869866141496));
#33680=CARTESIAN_POINT('Ctrl Pts',(0.700776341940978,3.8700647951392,37.681133355355));
#33681=CARTESIAN_POINT('Ctrl Pts',(0.814937234059428,3.84939298301038,37.6752734373361));
#33682=CARTESIAN_POINT('Ctrl Pts',(0.928102727263295,3.82368004145438,37.6694135193173));
#33683=CARTESIAN_POINT('Ctrl Pts',(1.03980362436862,3.79305911142311,37.6635536012984));
#33684=CARTESIAN_POINT('Ctrl Pts',(1.15157973289195,3.76241756344134,37.6576897376286));
#33685=CARTESIAN_POINT('Ctrl Pts',(1.2618888891731,3.72686157322117,37.6518258739589));
#33686=CARTESIAN_POINT('Ctrl Pts',(1.37027986241766,3.68657321894637,37.6459620102891));
#33687=CARTESIAN_POINT('Ctrl Pts',(1.47883073841939,3.64622542965834,37.64008949601));
#33688=CARTESIAN_POINT('Ctrl Pts',(1.5854574043302,3.6011315032136,37.6342169817309));
#33689=CARTESIAN_POINT('Ctrl Pts',(1.68973121106261,3.55152043980615,37.6283444674517));
#33690=CARTESIAN_POINT('Ctrl Pts',(1.7185502575496,3.53780900462016,37.6267214303026));
#33691=CARTESIAN_POINT('Ctrl Pts',(1.74718974257687,3.52375278791357,37.6250983931535));
#33692=CARTESIAN_POINT('Ctrl Pts',(1.7756410032213,3.50935721004278,37.6234753560044));
#33693=CARTESIAN_POINT('Ctrl Pts',(1.87857723493968,3.45727422651714,37.6176032320885));
#33694=CARTESIAN_POINT('Ctrl Pts',(1.97939255308003,3.40057110844653,37.6117311081726));
#33695=CARTESIAN_POINT('Ctrl Pts',(2.07764341029815,3.33944409440324,37.6058589842567));
#33696=CARTESIAN_POINT('Ctrl Pts',(2.17576688331402,3.27839633275672,37.5999944736669));
#33697=CARTESIAN_POINT('Ctrl Pts',(2.27133215960027,3.21293629767389,37.5941299630771));
#33698=CARTESIAN_POINT('Ctrl Pts',(2.36391832744339,3.14330703896028,37.5882654524874));
#33699=CARTESIAN_POINT('Ctrl Pts',(2.45640922502803,3.07374942807084,37.5824069764215));
#33700=CARTESIAN_POINT('Ctrl Pts',(2.54592678312613,3.00003137372826,37.5765485003556));
#33701=CARTESIAN_POINT('Ctrl Pts',(2.63207782173528,2.92243996351152,37.5706900242897));
#33702=CARTESIAN_POINT('Ctrl Pts',(2.72162591098664,2.84178902024491,37.5646005406793));
#33703=CARTESIAN_POINT('Ctrl Pts',(2.8075361396623,2.75695321399475,37.5585110570689));
#33704=CARTESIAN_POINT('Ctrl Pts',(2.88940329059112,2.66830238622259,37.5524215734586));
#33705=CARTESIAN_POINT('Ctrl Pts',(2.96807346463353,2.583113443274,37.5465698889915));
#33706=CARTESIAN_POINT('Ctrl Pts',(3.0430100991615,2.49440217895448,37.5407182045244));
#33707=CARTESIAN_POINT('Ctrl Pts',(3.11389077470868,2.4025347537932,37.5348665200573));
#33708=CARTESIAN_POINT('Ctrl Pts',(3.18476063940591,2.31068134041921,37.5290157280998));
#33709=CARTESIAN_POINT('Ctrl Pts',(3.25157552266725,2.21567305056715,37.5231649361423));
#33710=CARTESIAN_POINT('Ctrl Pts',(3.31405380919675,2.11790848474349,37.5173141441848));
#33711=CARTESIAN_POINT('Ctrl Pts',(3.3765376993061,2.02013515056877,37.5114628274789));
#33712=CARTESIAN_POINT('Ctrl Pts',(3.43468399686684,1.91960539737308,37.505611510773));
#33713=CARTESIAN_POINT('Ctrl Pts',(3.48825526576596,1.81674549699621,37.4997601940671));
#33714=CARTESIAN_POINT('Ctrl Pts',(3.54184431489582,1.71385145755939,37.4939069353172));
#33715=CARTESIAN_POINT('Ctrl Pts',(3.59085512516964,1.60862609961033,37.4880536765674));
#33716=CARTESIAN_POINT('Ctrl Pts',(3.63509724358918,1.501518241531,37.4822004178175));
#33717=CARTESIAN_POINT('Ctrl Pts',(3.67938969604625,1.39428852737559,37.4763404998443));
#33718=CARTESIAN_POINT('Ctrl Pts',(3.71890246993564,1.28517242061843,37.4704805818711));
#33719=CARTESIAN_POINT('Ctrl Pts',(3.75349406598325,1.17463666579437,37.464620663898));
#33720=CARTESIAN_POINT('Ctrl Pts',(3.78810895354121,1.06402648408717,37.4587568002745));
#33721=CARTESIAN_POINT('Ctrl Pts',(3.81779595965542,0.951995149594837,37.4528929366511));
#33722=CARTESIAN_POINT('Ctrl Pts',(3.84246447098273,0.839020732303683,37.4470290730277));
#33723=CARTESIAN_POINT('Ctrl Pts',(3.86716937429586,0.725879650581997,37.4411565587954));
#33724=CARTESIAN_POINT('Ctrl Pts',(3.88684093685391,0.611793115212634,37.4352840445631));
#33725=CARTESIAN_POINT('Ctrl Pts',(3.90144022942924,0.497245549191858,37.4294115303309));
#33726=CARTESIAN_POINT('Ctrl Pts',(3.9054751622212,0.465587047384892,37.4277884927676));
#33727=CARTESIAN_POINT('Ctrl Pts',(3.90912295559818,0.433893334164532,37.4261654552043));
#33728=CARTESIAN_POINT('Ctrl Pts',(3.9123834894837,0.402174627761775,37.424542417641));
#33729=CARTESIAN_POINT('Ctrl Pts',(3.92602993472042,0.269421034300653,37.417749452439));
#33730=CARTESIAN_POINT('Ctrl Pts',(3.93292115709448,0.135961246390276,37.410956487237));
#33731=CARTESIAN_POINT('Ctrl Pts',(3.93299932738369,0.00230017378215415,
37.404163522035));
#33732=CARTESIAN_POINT('',(-2.80846544028688,-2.75336355585568,38.));
#33733=CARTESIAN_POINT('Origin',(0.,0.,38.));
#33734=CARTESIAN_POINT('Ctrl Pts',(3.93299950757024,0.00196810879246953,
37.220836477965));
#33735=CARTESIAN_POINT('Ctrl Pts',(3.93294383452817,0.113223161314397,37.2264931957242));
#33736=CARTESIAN_POINT('Ctrl Pts',(3.92816790717577,0.22435667800964,37.2321499134834));
#33737=CARTESIAN_POINT('Ctrl Pts',(3.91869980905131,0.335083282992792,37.2378066312426));
#33738=CARTESIAN_POINT('Ctrl Pts',(3.90887116844884,0.450026325534738,37.2436787552018));
#33739=CARTESIAN_POINT('Ctrl Pts',(3.89396450975248,0.564729262387047,37.249550879161));
#33740=CARTESIAN_POINT('Ctrl Pts',(3.87399604281211,0.678707345087798,37.2554230031202));
#33741=CARTESIAN_POINT('Ctrl Pts',(3.85405346538562,0.79253765294116,37.261287513754));
#33742=CARTESIAN_POINT('Ctrl Pts',(3.82906220129585,0.905644572093272,37.2671520243879));
#33743=CARTESIAN_POINT('Ctrl Pts',(3.79909033948502,1.01754685023913,37.2730165350218));
#33744=CARTESIAN_POINT('Ctrl Pts',(3.76914931842163,1.12933398205476,37.2788750111326));
#33745=CARTESIAN_POINT('Ctrl Pts',(3.73423799979103,1.23991854148262,37.2847334872434));
#33746=CARTESIAN_POINT('Ctrl Pts',(3.69447568419538,1.34882853576318,37.2905919633542));
#33747=CARTESIAN_POINT('Ctrl Pts',(3.65314548775988,1.46203299556326,37.296681446948));
#33748=CARTESIAN_POINT('Ctrl Pts',(3.6065739399445,1.57342766445927,37.3027709305419));
#33749=CARTESIAN_POINT('Ctrl Pts',(3.55495259639291,1.6824984509352,37.3088604141357));
#33750=CARTESIAN_POINT('Ctrl Pts',(3.50534710653775,1.78730993819564,37.3147120986494));
#33751=CARTESIAN_POINT('Ctrl Pts',(3.45107901028721,1.88997522706534,37.3205637831631));
#33752=CARTESIAN_POINT('Ctrl Pts',(3.392367399822,1.99005839729012,37.3264154676768));
#33753=CARTESIAN_POINT('Ctrl Pts',(3.33366474415319,2.09012630265662,37.3322662596814));
#33754=CARTESIAN_POINT('Ctrl Pts',(3.27052013093913,2.1876125159477,37.338117051686));
#33755=CARTESIAN_POINT('Ctrl Pts',(3.20319799362034,2.28210683660223,37.3439678436907));
#33756=CARTESIAN_POINT('Ctrl Pts',(3.13586981827867,2.37660963231256,37.3498191604442));
#33757=CARTESIAN_POINT('Ctrl Pts',(3.06436361390616,2.46811966523383,37.3556704771977));
#33758=CARTESIAN_POINT('Ctrl Pts',(2.98898599387445,2.55625736740696,37.3615217939512));
#33759=CARTESIAN_POINT('Ctrl Pts',(2.91358335610828,2.64442432236928,37.3673750527492));
#33760=CARTESIAN_POINT('Ctrl Pts',(2.83430701626353,2.72921640696602,37.3732283115471));
#33761=CARTESIAN_POINT('Ctrl Pts',(2.75150206251009,2.81028920220014,37.3790815703451));
#33762=CARTESIAN_POINT('Ctrl Pts',(2.66860290196837,2.89145423355433,37.3849414883668));
#33763=CARTESIAN_POINT('Ctrl Pts',(2.58216741028541,2.96889124035578,37.3908014063884));
#33764=CARTESIAN_POINT('Ctrl Pts',(2.49257560162771,3.04229450746805,37.3966613244101));
#33765=CARTESIAN_POINT('Ctrl Pts',(2.4029234682402,3.11574719910163,37.4025251880824));
#33766=CARTESIAN_POINT('Ctrl Pts',(2.31011111636953,3.18516049589827,37.4083890517546));
#33767=CARTESIAN_POINT('Ctrl Pts',(2.21454808627185,3.25027164612278,37.4142529154269));
#33768=CARTESIAN_POINT('Ctrl Pts',(2.11884407772622,3.31547885095014,37.4201254297081));
#33769=CARTESIAN_POINT('Ctrl Pts',(2.02038164240613,3.37637102573865,37.4259979439892));
#33770=CARTESIAN_POINT('Ctrl Pts',(1.91959553306117,3.4327309812235,37.4318704582704));
#33771=CARTESIAN_POINT('Ctrl Pts',(1.89174041207018,3.44830766524553,37.4334934953822));
#33772=CARTESIAN_POINT('Ctrl Pts',(1.86370791579227,3.46353843799419,37.4351165324941));
#33773=CARTESIAN_POINT('Ctrl Pts',(1.83550747679674,3.47841936842343,37.4367395696059));
#33774=CARTESIAN_POINT('Ctrl Pts',(1.73347871087051,3.53225835184389,37.4426116935682));
#33775=CARTESIAN_POINT('Ctrl Pts',(1.62890808433844,3.5816947379408,37.4484838175304));
#33776=CARTESIAN_POINT('Ctrl Pts',(1.52221224378136,3.62648023362628,37.4543559414927));
#33777=CARTESIAN_POINT('Ctrl Pts',(1.41565473650146,3.67120766402677,37.4602204521296));
#33778=CARTESIAN_POINT('Ctrl Pts',(1.30697787232185,3.71129603691539,37.4660849627664));
#33779=CARTESIAN_POINT('Ctrl Pts',(1.19662338876077,3.74654260158225,37.4719494734033));
#33780=CARTESIAN_POINT('Ctrl Pts',(1.0863824588669,3.78175289788424,37.477807949517));
#33781=CARTESIAN_POINT('Ctrl Pts',(0.974467734634347,3.81213117071812,37.4836664256307));
#33782=CARTESIAN_POINT('Ctrl Pts',(0.861340834317039,3.83752276438043,37.4895249017444));
#33783=CARTESIAN_POINT('Ctrl Pts',(0.743753190362223,3.86391558223926,37.4956143853371));
#33784=CARTESIAN_POINT('Ctrl Pts',(0.624856227806823,3.88492019147547,37.5017038689298));
#33785=CARTESIAN_POINT('Ctrl Pts',(0.505186031405749,3.90041998683123,37.5077933525225));
#33786=CARTESIAN_POINT('Ctrl Pts',(0.390189049364761,3.91531450310821,37.5136450370389));
#33787=CARTESIAN_POINT('Ctrl Pts',(0.274478539588281,3.92512601396187,37.5194967215552));
#33788=CARTESIAN_POINT('Ctrl Pts',(0.158539689569357,3.9298033241921,37.5253484060716));
#33789=CARTESIAN_POINT('Ctrl Pts',(0.0426185227462051,3.9344799210308,37.5311991980788));
#33790=CARTESIAN_POINT('Ctrl Pts',(-0.0735305021100036,3.93402385758884,
37.537049990086));
#33791=CARTESIAN_POINT('Ctrl Pts',(-0.189419339084341,3.92843598827585,
37.5429007820933));
#33792=CARTESIAN_POINT('Ctrl Pts',(-0.305318569954967,3.92284761779523,
37.5487520988493));
#33793=CARTESIAN_POINT('Ctrl Pts',(-0.420957153596696,3.91212654639289,
37.5546034156052));
#33794=CARTESIAN_POINT('Ctrl Pts',(-0.535850027816559,3.89632567269331,
37.5604547323612));
#33795=CARTESIAN_POINT('Ctrl Pts',(-0.650781034830726,3.88051955470447,
37.5663079911616));
#33796=CARTESIAN_POINT('Ctrl Pts',(-0.76496543094427,3.85963033825317,37.572161249962));
#33797=CARTESIAN_POINT('Ctrl Pts',(-0.877926940000475,3.83376228892995,
37.5780145087623));
#33798=CARTESIAN_POINT('Ctrl Pts',(-0.991016964806267,3.80786480965508,
37.5838744267862));
#33799=CARTESIAN_POINT('Ctrl Pts',(-1.10288092238968,3.77697728386623,37.5897343448101));
#33800=CARTESIAN_POINT('Ctrl Pts',(-1.21305623145749,3.74125427889126,37.595594262834));
#33801=CARTESIAN_POINT('Ctrl Pts',(-1.3233057247134,3.70550722059488,37.6014581265084));
#33802=CARTESIAN_POINT('Ctrl Pts',(-1.43186391914719,3.66491834447394,37.6073219901828));
#33803=CARTESIAN_POINT('Ctrl Pts',(-1.53828843031218,3.61969027751929,37.6131858538572));
#33804=CARTESIAN_POINT('Ctrl Pts',(-1.64486994321869,3.57439548829174,37.6190583681404));
#33805=CARTESIAN_POINT('Ctrl Pts',(-1.74931111907896,3.52444802672684,37.6249308824235));
#33806=CARTESIAN_POINT('Ctrl Pts',(-1.85119428810024,3.47009635423932,37.6308033967067));
#33807=CARTESIAN_POINT('Ctrl Pts',(-1.87935261244782,3.45507471683406,37.6324264337942));
#33808=CARTESIAN_POINT('Ctrl Pts',(-1.90731571692631,3.43971691608275,37.6340494708818));
#33809=CARTESIAN_POINT('Ctrl Pts',(-1.93507519692215,3.42402876481152,37.6356725079694));
#33810=CARTESIAN_POINT('Ctrl Pts',(-2.03550858192254,3.36726926727036,37.6415446319685));
#33811=CARTESIAN_POINT('Ctrl Pts',(-2.13361092601821,3.30599200839285,37.6474167559676));
#33812=CARTESIAN_POINT('Ctrl Pts',(-2.22894817098408,3.24041340743226,37.6532888799667));
#33813=CARTESIAN_POINT('Ctrl Pts',(-2.32416180932104,3.17491983042843,37.6591533906405));
#33814=CARTESIAN_POINT('Ctrl Pts',(-2.41661714034022,3.10513623365194,37.6650179013144));
#33815=CARTESIAN_POINT('Ctrl Pts',(-2.50590486924698,3.03132475764051,37.6708824119883));
#33816=CARTESIAN_POINT('Ctrl Pts',(-2.59510072197035,2.95758923290243,37.6767408881391));
#33817=CARTESIAN_POINT('Ctrl Pts',(-2.6811351390289,2.87983433464965,37.6825993642899));
#33818=CARTESIAN_POINT('Ctrl Pts',(-2.76362855226727,2.79836491992969,37.6884578404407));
#33819=CARTESIAN_POINT('Ctrl Pts',(-2.84937478940238,2.71368305892279,37.6945473240195));
#33820=CARTESIAN_POINT('Ctrl Pts',(-2.93129464984765,2.62498797621149,37.7006368075984));
#33821=CARTESIAN_POINT('Ctrl Pts',(-3.00900034488857,2.53266774853325,37.7067262911772));
#33822=CARTESIAN_POINT('Ctrl Pts',(-3.08367157267096,2.44395269687256,37.7125779757308));
#33823=CARTESIAN_POINT('Ctrl Pts',(-3.15445130019248,2.3518906626465,37.7184296602843));
#33824=CARTESIAN_POINT('Ctrl Pts',(-3.22103427970653,2.25686223969374,37.7242813448378));
#33825=CARTESIAN_POINT('Ctrl Pts',(-3.28760710386799,2.16184831064238,37.7301321368822));
#33826=CARTESIAN_POINT('Ctrl Pts',(-3.3499842155701,2.06386923093621,37.7359829289266));
#33827=CARTESIAN_POINT('Ctrl Pts',(-3.40790261924258,1.96333612449819,37.741833720971));
#33828=CARTESIAN_POINT('Ctrl Pts',(-3.46582621752925,1.86279400139762,37.747685037764));
#33829=CARTESIAN_POINT('Ctrl Pts',(-3.51929010644619,1.75969775444043,37.7535363545571));
#33830=CARTESIAN_POINT('Ctrl Pts',(-3.5680766948491,1.65448411889468,37.7593876713502));
#33831=CARTESIAN_POINT('Ctrl Pts',(-3.61687947545567,1.54923556308354,37.7652409301875));
#33832=CARTESIAN_POINT('Ctrl Pts',(-3.66100169490512,1.44186859615042,37.7710941890248));
#33833=CARTESIAN_POINT('Ctrl Pts',(-3.700273731881,1.33284031644884,37.7769474478621));
#33834=CARTESIAN_POINT('Ctrl Pts',(-3.73959044845629,1.22368799582054,37.7828073659227));
#33835=CARTESIAN_POINT('Ctrl Pts',(-3.77404582853623,1.11287097908174,37.7886672839832));
#33836=CARTESIAN_POINT('Ctrl Pts',(-3.80351997677793,1.00086202158501,37.7945272020437));
#33837=CARTESIAN_POINT('Ctrl Pts',(-3.83301397080609,0.888777645255649,
37.8003910657546));
#33838=CARTESIAN_POINT('Ctrl Pts',(-3.85751996731369,0.775500133178225,
37.8062549294654));
#33839=CARTESIAN_POINT('Ctrl Pts',(-3.87696942368802,0.661511215164319,
37.8121187931763));
#33840=CARTESIAN_POINT('Ctrl Pts',(-3.89644757268481,0.547354136101277,
37.8179913074954));
#33841=CARTESIAN_POINT('Ctrl Pts',(-3.91085424229471,0.432483965168503,
37.8238638218144));
#33842=CARTESIAN_POINT('Ctrl Pts',(-3.92017281141304,0.317386402761613,
37.8297363361335));
#33843=CARTESIAN_POINT('Ctrl Pts',(-3.92274826362267,0.285575910436055,
37.8313593728667));
#33844=CARTESIAN_POINT('Ctrl Pts',(-3.92493536749216,0.253748039177028,
37.8329824095998));
#33845=CARTESIAN_POINT('Ctrl Pts',(-3.92673447276226,0.221913001918477,
37.8346054463329));
#33846=CARTESIAN_POINT('Ctrl Pts',(-3.93324439359981,0.106720424887167,
37.8404782770253));
#33847=CARTESIAN_POINT('Ctrl Pts',(-3.93469208920761,-0.00895199463281238,
37.8463511077176));
#33848=CARTESIAN_POINT('Ctrl Pts',(-3.93102510557173,-0.124621905637643,
37.85222393841));
#33849=CARTESIAN_POINT('Ctrl Pts',(-3.92718047745846,-0.245895365207376,
37.8583812743096));
#33850=CARTESIAN_POINT('Ctrl Pts',(-3.91771306451741,-0.36716563417689,
37.8645386102092));
#33851=CARTESIAN_POINT('Ctrl Pts',(-3.90262370181262,-0.487870107764704,
37.8706959461088));
#33852=CARTESIAN_POINT('Ctrl Pts',(-3.88826876487249,-0.602699682786761,
37.876553593664));
#33853=CARTESIAN_POINT('Ctrl Pts',(-3.86882626391864,-0.717016759625243,
37.8824112412192));
#33854=CARTESIAN_POINT('Ctrl Pts',(-3.84435019811851,-0.830337614603938,
37.8882688887744));
#33855=CARTESIAN_POINT('Ctrl Pts',(-3.81989064215858,-0.943582031268476,
37.8941225851708));
#33856=CARTESIAN_POINT('Ctrl Pts',(-3.79040435949656,-1.05583115968554,
37.8999762815671));
#33857=CARTESIAN_POINT('Ctrl Pts',(-3.75599681193477,-1.16660916708889,
37.9058299779635));
#33858=CARTESIAN_POINT('Ctrl Pts',(-3.72160413907796,-1.27733928412237,
37.911681143752));
#33859=CARTESIAN_POINT('Ctrl Pts',(-3.68229455560271,-1.38659915110984,
37.9175323095406));
#33860=CARTESIAN_POINT('Ctrl Pts',(-3.63822380843997,-1.49392654427871,
37.9233834753292));
#33861=CARTESIAN_POINT('Ctrl Pts',(-3.59416143914316,-1.60123353446901,
37.9292335288089));
#33862=CARTESIAN_POINT('Ctrl Pts',(-3.54533986516638,-1.70660840017188,
37.9350835822886));
#33863=CARTESIAN_POINT('Ctrl Pts',(-3.49196329098949,-1.80960807203711,
37.9409336357683));
#33864=CARTESIAN_POINT('Ctrl Pts',(-3.43856616530903,-1.91264740171395,
37.9467859416855));
#33865=CARTESIAN_POINT('Ctrl Pts',(-3.38061072430561,-2.01330934241119,
37.9526382476027));
#33866=CARTESIAN_POINT('Ctrl Pts',(-3.31834743433787,-2.1111748636774,37.9584905535198));
#33867=CARTESIAN_POINT('Ctrl Pts',(-3.25607013218143,-2.20906240932026,
37.964344176483));
#33868=CARTESIAN_POINT('Ctrl Pts',(-3.18948328170545,-2.30415193962538,
37.9701977994461));
#33869=CARTESIAN_POINT('Ctrl Pts',(-3.1188803022657,-2.39605397688346,37.9760514224093));
#33870=CARTESIAN_POINT('Ctrl Pts',(-3.04821565354052,-2.48803628742478,
37.9819101583116));
#33871=CARTESIAN_POINT('Ctrl Pts',(-2.97352813414324,-2.57682522667805,
37.987768894214));
#33872=CARTESIAN_POINT('Ctrl Pts',(-2.89515090838893,-2.66206502881781,
37.9936276301164));
#33873=CARTESIAN_POINT('Ctrl Pts',(-2.86673472889935,-2.69296928058161,
37.995751753411));
#33874=CARTESIAN_POINT('Ctrl Pts',(-2.83783389725777,-2.72340736054617,
37.9978758767055));
#33875=CARTESIAN_POINT('Ctrl Pts',(-2.80846544028688,-2.75336355585568,
38.));
#33876=CARTESIAN_POINT('Origin',(0.,0.,32.));
#33877=CARTESIAN_POINT('',(3.93133412486678,0.00259602383233126,35.9708370172092));
#33878=CARTESIAN_POINT('',(3.93121085245411,0.00231623353798856,36.1541640353064));
#33879=CARTESIAN_POINT('',(3.933,4.81653586104654E-16,32.));
#33880=CARTESIAN_POINT('',(0.65368646409381,3.87829640520945,35.));
#33881=CARTESIAN_POINT('Ctrl Pts',(0.65368646409381,3.87829640520945,35.));
#33882=CARTESIAN_POINT('Ctrl Pts',(0.539330922767402,3.89757102005291,35.0058615808379));
#33883=CARTESIAN_POINT('Ctrl Pts',(0.424217848923065,3.91176742009041,35.0117231616759));
#33884=CARTESIAN_POINT('Ctrl Pts',(0.308833568652951,3.92085587938056,35.0175847425138));
#33885=CARTESIAN_POINT('Ctrl Pts',(0.193261297999275,3.92995914608592,35.02345587336));
#33886=CARTESIAN_POINT('Ctrl Pts',(0.0774173514306077,3.9339378322415,35.0293270042062));
#33887=CARTESIAN_POINT('Ctrl Pts',(-0.0382115899189808,3.93281437070145,
35.0351981350524));
#33888=CARTESIAN_POINT('Ctrl Pts',(-0.132391795727835,3.93189930706924,
35.0399801931165));
#33889=CARTESIAN_POINT('Ctrl Pts',(-0.226429308324548,3.92760039491556,
35.0447622511807));
#33890=CARTESIAN_POINT('Ctrl Pts',(-0.320064996648115,3.91995502498698,
35.0495443092448));
#33891=CARTESIAN_POINT('Ctrl Pts',(-0.435044857224395,3.91056689975203,
35.0554164332108));
#33892=CARTESIAN_POINT('Ctrl Pts',(-0.549804072018368,3.89609987364649,
35.0612885571768));
#33893=CARTESIAN_POINT('Ctrl Pts',(-0.663857834012495,3.87656829892371,
35.0671606811429));
#33894=CARTESIAN_POINT('Ctrl Pts',(-0.777763723039442,3.85706204727539,
35.0730251917836));
#33895=CARTESIAN_POINT('Ctrl Pts',(-0.890965574426317,3.83250437410963,
35.0788897024243));
#33896=CARTESIAN_POINT('Ctrl Pts',(-1.00298187849455,3.80296152378795,35.084754213065));
#33897=CARTESIAN_POINT('Ctrl Pts',(-1.11488291890037,3.77344907276532,35.0906126891826));
#33898=CARTESIAN_POINT('Ctrl Pts',(-1.22560044112233,3.73896175259171,35.0964711653002));
#33899=CARTESIAN_POINT('Ctrl Pts',(-1.33466199872459,3.69961705439367,35.1023296414178));
#33900=CARTESIAN_POINT('Ctrl Pts',(-1.44802399800991,3.65872094262829,35.108419125009));
#33901=CARTESIAN_POINT('Ctrl Pts',(-1.55959630369201,3.61257658314203,35.1145086086003));
#33902=CARTESIAN_POINT('Ctrl Pts',(-1.66886409402027,3.56137356025592,35.1205980921916));
#33903=CARTESIAN_POINT('Ctrl Pts',(-1.77386489214357,3.51217005524117,35.126449776712));
#33904=CARTESIAN_POINT('Ctrl Pts',(-1.87673737398393,3.45829575416629,35.1323014612324));
#33905=CARTESIAN_POINT('Ctrl Pts',(-1.97704478296076,3.39996807722773,35.1381531457528));
#33906=CARTESIAN_POINT('Ctrl Pts',(-2.07733689287734,3.34164929652778,35.1440039377641));
#33907=CARTESIAN_POINT('Ctrl Pts',(-2.17506435053188,3.27887869825674,35.1498547297754));
#33908=CARTESIAN_POINT('Ctrl Pts',(-2.26981594510763,3.21191914209171,35.1557055217867));
#33909=CARTESIAN_POINT('Ctrl Pts',(-2.36457603781286,3.14495358042376,35.1615568385468));
#33910=CARTESIAN_POINT('Ctrl Pts',(-2.45635939922802,3.07379855260523,35.167408155307));
#33911=CARTESIAN_POINT('Ctrl Pts',(-2.54478528928676,2.99875921531384,35.1732594720671));
#33912=CARTESIAN_POINT('Ctrl Pts',(-2.63324052778291,2.92369497256443,35.1791127308716));
#33913=CARTESIAN_POINT('Ctrl Pts',(-2.71833576408511,2.84474412420826,35.1849659896761));
#33914=CARTESIAN_POINT('Ctrl Pts',(-2.79972525940178,2.76225043612407,35.1908192484807));
#33915=CARTESIAN_POINT('Ctrl Pts',(-2.88120735114467,2.67966289537901,35.1966791665088));
#33916=CARTESIAN_POINT('Ctrl Pts',(-2.95897499634738,2.59352476425835,35.2025390845369));
#33917=CARTESIAN_POINT('Ctrl Pts',(-3.03272102596396,2.50421488268801,35.208399002565));
#33918=CARTESIAN_POINT('Ctrl Pts',(-3.10651671089285,2.4148448662184,35.2142628662436));
#33919=CARTESIAN_POINT('Ctrl Pts',(-3.1762851400794,2.32229917614978,35.2201267299223));
#33920=CARTESIAN_POINT('Ctrl Pts',(-3.24176199442419,2.22698634290983,35.2259905936009));
#33921=CARTESIAN_POINT('Ctrl Pts',(-3.3073354428715,2.13153290032515,35.2318631078883));
#33922=CARTESIAN_POINT('Ctrl Pts',(-3.36860446279633,2.03330451671135,35.2377356221756));
#33923=CARTESIAN_POINT('Ctrl Pts',(-3.42535020062493,1.93273510939258,35.243608136463));
#33924=CARTESIAN_POINT('Ctrl Pts',(-3.44103350599065,1.90493988131405,35.2452311735114));
#33925=CARTESIAN_POINT('Ctrl Pts',(-3.45637158232295,1.8769659537885,35.2468542105598));
#33926=CARTESIAN_POINT('Ctrl Pts',(-3.47136046246102,1.8488227442517,35.2484772476082));
#33927=CARTESIAN_POINT('Ctrl Pts',(-3.52559000846581,1.74700102960462,35.2543493715742));
#33928=CARTESIAN_POINT('Ctrl Pts',(-3.57542672946076,1.6426206029676,35.2602214955402));
#33929=CARTESIAN_POINT('Ctrl Pts',(-3.62062073765856,1.53609715644447,35.2660936195063));
#33930=CARTESIAN_POINT('Ctrl Pts',(-3.66575615092748,1.4297118196846,35.271958130147));
#33931=CARTESIAN_POINT('Ctrl Pts',(-3.70626066176825,1.32118936546262,35.2778226407877));
#33932=CARTESIAN_POINT('Ctrl Pts',(-3.74192982829283,1.21097075114654,35.2836871514284));
#33933=CARTESIAN_POINT('Ctrl Pts',(-3.77756229159994,1.10086555068798,35.289545627546));
#33934=CARTESIAN_POINT('Ctrl Pts',(-3.80836918061562,0.989068052643565,
35.2954041036637));
#33935=CARTESIAN_POINT('Ctrl Pts',(-3.8341940719254,0.876039279263296,35.3012625797813));
#33936=CARTESIAN_POINT('Ctrl Pts',(-3.86103727290798,0.758553631627159,
35.3073520633725));
#33937=CARTESIAN_POINT('Ctrl Pts',(-3.88249732192508,0.639738028258825,
35.3134415469638));
#33938=CARTESIAN_POINT('Ctrl Pts',(-3.89845556038526,0.52012810316428,35.3195310305551));
#33939=CARTESIAN_POINT('Ctrl Pts',(-3.91379061722067,0.405189038681629,
35.3253827150755));
#33940=CARTESIAN_POINT('Ctrl Pts',(-3.92404544006576,0.289516974445092,
35.3312343995959));
#33941=CARTESIAN_POINT('Ctrl Pts',(-3.92916697493633,0.173596898214589,
35.3370860841163));
#33942=CARTESIAN_POINT('Ctrl Pts',(-3.9342877286615,0.0576945023155024,
35.3429368761276));
#33943=CARTESIAN_POINT('Ctrl Pts',(-3.93427673289576,-0.0584554174693667,
35.3487876681389));
#33944=CARTESIAN_POINT('Ctrl Pts',(-3.92913297192955,-0.174364815533547,
35.3546384601502));
#33945=CARTESIAN_POINT('Ctrl Pts',(-3.92398874962709,-0.290284609338774,
35.3604897769103));
#33946=CARTESIAN_POINT('Ctrl Pts',(-3.91371086531983,-0.405963425509345,
35.3663410936704));
#33947=CARTESIAN_POINT('Ctrl Pts',(-3.89835035856407,-0.520916002713838,
35.3721924104306));
#33948=CARTESIAN_POINT('Ctrl Pts',(-3.88298475367618,-0.635906732528653,
35.3780456692351));
#33949=CARTESIAN_POINT('Ctrl Pts',(-3.86253322674438,-0.750170334535612,
35.3838989280396));
#33950=CARTESIAN_POINT('Ctrl Pts',(-3.8370982175806,-0.863230136545143,
35.3897521868441));
#33951=CARTESIAN_POINT('Ctrl Pts',(-3.81163427113265,-0.976418566132486,
35.3956121048722));
#33952=CARTESIAN_POINT('Ctrl Pts',(-3.78117561670702,-1.08840005854956,
35.4014720229003));
#33953=CARTESIAN_POINT('Ctrl Pts',(-3.74587504796018,-1.19871144362158,
35.4073319409285));
#33954=CARTESIAN_POINT('Ctrl Pts',(-3.71055071033013,-1.3090971045062,35.4131958046071));
#33955=CARTESIAN_POINT('Ctrl Pts',(-3.67037810963136,-1.41781003204734,
35.4190596682857));
#33956=CARTESIAN_POINT('Ctrl Pts',(-3.62555817622155,-1.52440706861163,
35.4249235319644));
#33957=CARTESIAN_POINT('Ctrl Pts',(-3.58067212263409,-1.6311613614335,35.4307960462517));
#33958=CARTESIAN_POINT('Ctrl Pts',(-3.53112522943475,-1.73579316120889,
35.4366685605391));
#33959=CARTESIAN_POINT('Ctrl Pts',(-3.47716435577114,-1.8378838491468,35.4425410748265));
#33960=CARTESIAN_POINT('Ctrl Pts',(-3.46225072715634,-1.86609952657313,
35.4441641118749));
#33961=CARTESIAN_POINT('Ctrl Pts',(-3.44700018962873,-1.89412127369666,
35.4457871489232));
#33962=CARTESIAN_POINT('Ctrl Pts',(-3.43141852376622,-1.92194066369231,
35.4474101859715));
#33963=CARTESIAN_POINT('Ctrl Pts',(-3.37504428780202,-2.0225908040453,35.4532823099376));
#33964=CARTESIAN_POINT('Ctrl Pts',(-3.31414339153919,-2.12092723197976,
35.4591544339036));
#33965=CARTESIAN_POINT('Ctrl Pts',(-3.24893058939597,-2.21651506317623,
35.4650265578697));
#33966=CARTESIAN_POINT('Ctrl Pts',(-3.18380233694565,-2.31197896285149,
35.4708910685104));
#33967=CARTESIAN_POINT('Ctrl Pts',(-3.11437352686747,-2.40470101416566,
35.4767555791511));
#33968=CARTESIAN_POINT('Ctrl Pts',(-3.04090472941805,-2.49427092085101,
35.4826200897918));
#33969=CARTESIAN_POINT('Ctrl Pts',(-2.96751153063028,-2.58374866099349,
35.4884785659094));
#33970=CARTESIAN_POINT('Ctrl Pts',(-2.89008687375796,-2.67008039031691,
35.494337042027));
#33971=CARTESIAN_POINT('Ctrl Pts',(-2.80893415916184,-2.75288537529149,
35.5001955181447));
#33972=CARTESIAN_POINT('Ctrl Pts',(-2.72458148553147,-2.83895547051,35.5062850017359));
#33973=CARTESIAN_POINT('Ctrl Pts',(-2.63620095757036,-2.92121459514035,
35.5123744853272));
#33974=CARTESIAN_POINT('Ctrl Pts',(-2.54417916322711,-2.99927347626071,
35.5184639689185));
#33975=CARTESIAN_POINT('Ctrl Pts',(-2.45575089153084,-3.0742840973563,35.5243156534389));
#33976=CARTESIAN_POINT('Ctrl Pts',(-2.36396075026656,-3.14541607190399,
35.5301673379593));
#33977=CARTESIAN_POINT('Ctrl Pts',(-2.26918816081457,-3.21236269602593,
35.5360190224797));
#33978=CARTESIAN_POINT('Ctrl Pts',(-2.17443002624266,-3.27929910933239,
35.541869814491));
#33979=CARTESIAN_POINT('Ctrl Pts',(-2.07669068551382,-3.34205120300941,
35.5477206065023));
#33980=CARTESIAN_POINT('Ctrl Pts',(-1.97638025177208,-3.40035440805886,
35.5535713985136));
#33981=CARTESIAN_POINT('Ctrl Pts',(-1.87606082133687,-3.45866284223598,
35.5594227152738));
#33982=CARTESIAN_POINT('Ctrl Pts',(-1.77317019692764,-3.51252138682477,
35.5652740320339));
#33983=CARTESIAN_POINT('Ctrl Pts',(-1.66814427682793,-3.5617107787812,35.5711253487941));
#33984=CARTESIAN_POINT('Ctrl Pts',(-1.56308349876298,-3.61091649663237,
35.5769786075986));
#33985=CARTESIAN_POINT('Ctrl Pts',(-1.45588638998729,-3.65544980515002,
35.5828318664031));
#33986=CARTESIAN_POINT('Ctrl Pts',(-1.34700939553298,-3.69513933273779,
35.5886851252076));
#33987=CARTESIAN_POINT('Ctrl Pts',(-1.23800853226013,-3.73487401490496,
35.5945450432357));
#33988=CARTESIAN_POINT('Ctrl Pts',(-1.12732435725081,-3.76975377516615,
35.6004049612638));
#33989=CARTESIAN_POINT('Ctrl Pts',(-1.01542916296309,-3.79965690753837,
35.6062648792919));
#33990=CARTESIAN_POINT('Ctrl Pts',(-0.903458626439311,-3.82958017454527,
35.6121287429706));
#33991=CARTESIAN_POINT('Ctrl Pts',(-0.790275849730697,-3.85452005260933,
35.6179926066492));
#33992=CARTESIAN_POINT('Ctrl Pts',(-0.676362296463616,-3.87440615371214,
35.6238564703278));
#33993=CARTESIAN_POINT('Ctrl Pts',(-0.562280693316787,-3.89432159159536,
35.6297289846152));
#33994=CARTESIAN_POINT('Ctrl Pts',(-0.447466570445664,-3.90916831983273,
35.6356014989026));
#33995=CARTESIAN_POINT('Ctrl Pts',(-0.33240556098613,-3.91892785631804,
35.64147401319));
#33996=CARTESIAN_POINT('Ctrl Pts',(-0.300605164761025,-3.92162518296817,
35.6430970502384));
#33997=CARTESIAN_POINT('Ctrl Pts',(-0.268785901634046,-3.92393423057186,
35.6447200872867));
#33998=CARTESIAN_POINT('Ctrl Pts',(-0.236957985810335,-3.92585530973324,
35.6463431243351));
#33999=CARTESIAN_POINT('Ctrl Pts',(-0.12180505847427,-3.93280574564311,
35.6522152483011));
#34000=CARTESIAN_POINT('Ctrl Pts',(-0.00615301487706181,-3.93469705103759,
35.6580873722671));
#34001=CARTESIAN_POINT('Ctrl Pts',(0.109516173067406,-3.93147494050727,
35.6639594962331));
#34002=CARTESIAN_POINT('Ctrl Pts',(0.225035393613353,-3.92825700750722,
35.6698240068738));
#34003=CARTESIAN_POINT('Ctrl Pts',(0.340571304870519,-3.9199388539467,35.6756885175145));
#34004=CARTESIAN_POINT('Ctrl Pts',(0.455637867855379,-3.90651803187649,
35.6815530281552));
#34005=CARTESIAN_POINT('Ctrl Pts',(0.570586028491408,-3.89311101969871,
35.6874115042727));
#34006=CARTESIAN_POINT('Ctrl Pts',(0.685065393318412,-3.87461183029995,
35.6932699803903));
#34007=CARTESIAN_POINT('Ctrl Pts',(0.798591655527019,-3.85107002892996,
35.6991284565079));
#34008=CARTESIAN_POINT('Ctrl Pts',(0.91659440863619,-3.8265999431475,35.7052179400992));
#34009=CARTESIAN_POINT('Ctrl Pts',(1.03356689370182,-3.79668140298861,35.7113074236904));
#34010=CARTESIAN_POINT('Ctrl Pts',(1.14897266828838,-3.76142935697672,35.7173969072817));
#34011=CARTESIAN_POINT('Ctrl Pts',(1.25987175760961,-3.7275539307822,35.7232485918021));
#34012=CARTESIAN_POINT('Ctrl Pts',(1.36932377014749,-3.68875386908664,35.7291002763224));
#34013=CARTESIAN_POINT('Ctrl Pts',(1.47686561295159,-3.64518270615906,35.7349519608428));
#34014=CARTESIAN_POINT('Ctrl Pts',(1.58439105328696,-3.60161818878097,35.7408027528541));
#34015=CARTESIAN_POINT('Ctrl Pts',(1.69000652011514,-3.55328417225595,35.7466535448653));
#34016=CARTESIAN_POINT('Ctrl Pts',(1.79326779031035,-3.50038278367315,35.7525043368766));
#34017=CARTESIAN_POINT('Ctrl Pts',(1.89653832185472,-3.4474766504438,35.7583556536367));
#34018=CARTESIAN_POINT('Ctrl Pts',(1.99745386907001,-3.39000251933694,35.7642069703967));
#34019=CARTESIAN_POINT('Ctrl Pts',(2.09559439821291,-3.32820869510592,35.7700582871568));
#34020=CARTESIAN_POINT('Ctrl Pts',(2.19376750006895,-3.26639436158554,35.7759115459613));
#34021=CARTESIAN_POINT('Ctrl Pts',(2.28916340279892,-3.2002577042806,35.7817648047657));
#34022=CARTESIAN_POINT('Ctrl Pts',(2.38139126813706,-3.13009019487308,35.7876180635702));
#34023=CARTESIAN_POINT('Ctrl Pts',(2.4737240606623,-3.05984285623649,35.7934779815983));
#34024=CARTESIAN_POINT('Ctrl Pts',(2.56288129257514,-2.98555576266775,35.7993378996263));
#34025=CARTESIAN_POINT('Ctrl Pts',(2.64850535321294,-2.90756055723736,35.8051978176544));
#34026=CARTESIAN_POINT('Ctrl Pts',(2.73418706698117,-2.82951283540307,35.811061681333));
#34027=CARTESIAN_POINT('Ctrl Pts',(2.81633058015491,-2.74775232106522,35.8169255450116));
#34028=CARTESIAN_POINT('Ctrl Pts',(2.89461650753271,-2.66264610384466,35.8227894086902));
#34029=CARTESIAN_POINT('Ctrl Pts',(2.9730179254756,-2.57741433449169,35.8286619229776));
#34030=CARTESIAN_POINT('Ctrl Pts',(3.04755013455306,-2.48882732664115,35.834534437265));
#34031=CARTESIAN_POINT('Ctrl Pts',(3.11793517238354,-2.39728372555558,35.8404069515523));
#34032=CARTESIAN_POINT('Ctrl Pts',(3.13738808786115,-2.37198303681087,35.842029988601));
#34033=CARTESIAN_POINT('Ctrl Pts',(3.15652448380116,-2.34645666696298,35.8436530256498));
#34034=CARTESIAN_POINT('Ctrl Pts',(3.17533910233628,-2.32071337850546,35.8452760626985));
#34035=CARTESIAN_POINT('Ctrl Pts',(3.24386965336691,-2.22694577221349,35.8511878287586));
#34036=CARTESIAN_POINT('Ctrl Pts',(3.30835742877721,-2.12998392340895,35.8570995948188));
#34037=CARTESIAN_POINT('Ctrl Pts',(3.36849264223259,-2.03020844230953,35.8630113608789));
#34038=CARTESIAN_POINT('Ctrl Pts',(3.42854818206181,-1.9305651545445,35.8689152943929));
#34039=CARTESIAN_POINT('Ctrl Pts',(3.48426242031965,-1.82811599172916,35.8748192279068));
#34040=CARTESIAN_POINT('Ctrl Pts',(3.53536685330977,-1.72327311025228,35.8807231614208));
#34041=CARTESIAN_POINT('Ctrl Pts',(3.58641539569186,-1.61854489069514,35.8866206380695));
#34042=CARTESIAN_POINT('Ctrl Pts',(3.63286398405451,-1.51142852206661,35.8925181147183));
#34043=CARTESIAN_POINT('Ctrl Pts',(3.67448867569264,-1.40236299587752,35.898415591367));
#34044=CARTESIAN_POINT('Ctrl Pts',(3.71708453564452,-1.29075280259325,35.9044506652502));
#34045=CARTESIAN_POINT('Ctrl Pts',(3.75462837515732,-1.17710173246275,35.9104857391334));
#34046=CARTESIAN_POINT('Ctrl Pts',(3.78693102001708,-1.06190510387342,35.9165208130165));
#34047=CARTESIAN_POINT('Ctrl Pts',(3.81844890924432,-0.949507044984043,
35.9224092717156));
#34048=CARTESIAN_POINT('Ctrl Pts',(3.84497722627513,-0.835638076692662,
35.9282977304147));
#34049=CARTESIAN_POINT('Ctrl Pts',(3.8663899645524,-0.720775722405051,35.9341861891138));
#34050=CARTESIAN_POINT('Ctrl Pts',(3.88860242803569,-0.601623476803267,
35.940294570589));
#34051=CARTESIAN_POINT('Ctrl Pts',(3.90530960984758,-0.481402630182505,
35.9464029520642));
#34052=CARTESIAN_POINT('Ctrl Pts',(3.91642873442305,-0.360659074730551,
35.9525113335394));
#34053=CARTESIAN_POINT('Ctrl Pts',(3.92754785899851,-0.239915519278558,
35.9586197150147));
#34054=CARTESIAN_POINT('Ctrl Pts',(3.93307887719384,-0.118649740920967,
35.9647280964899));
#34055=CARTESIAN_POINT('Ctrl Pts',(3.93299914955306,0.00258642898096291,
35.9708364779651));
#34056=CARTESIAN_POINT('',(3.48437472100057,1.8241770209199,35.));
#34057=CARTESIAN_POINT('Origin',(0.,0.,35.));
#34058=CARTESIAN_POINT('Ctrl Pts',(3.93299932332396,0.0023071049629667,
36.154163522035));
#34059=CARTESIAN_POINT('Ctrl Pts',(3.93306815257745,-0.11502843536642,36.1482539137099));
#34060=CARTESIAN_POINT('Ctrl Pts',(3.92788182847184,-0.232374625365518,
36.1423443053847));
#34061=CARTESIAN_POINT('Ctrl Pts',(3.91746406086123,-0.349233921406056,
36.1364346970596));
#34062=CARTESIAN_POINT('Ctrl Pts',(3.90704445346722,-0.466113854861418,
36.1305240450945));
#34063=CARTESIAN_POINT('Ctrl Pts',(3.89139159917373,-0.582506322944185,
36.1246133931293));
#34064=CARTESIAN_POINT('Ctrl Pts',(3.87058107839869,-0.697919132523272,
36.1187027411642));
#34065=CARTESIAN_POINT('Ctrl Pts',(3.84976222824505,-0.813378135899996,
36.1127897234698));
#34066=CARTESIAN_POINT('Ctrl Pts',(3.82378167424935,-0.927856305137044,
36.1068767057753));
#34067=CARTESIAN_POINT('Ctrl Pts',(3.79276595892408,-1.04087241332774,36.1009636880809));
#34068=CARTESIAN_POINT('Ctrl Pts',(3.76170851327563,-1.15404057987561,36.0950427146732));
#34069=CARTESIAN_POINT('Ctrl Pts',(3.72560248091587,-1.26574236800933,36.0891217412655));
#34070=CARTESIAN_POINT('Ctrl Pts',(3.68462423432077,-1.37551199626033,36.0832007678578));
#34071=CARTESIAN_POINT('Ctrl Pts',(3.64361753378841,-1.48535784490568,36.0772756831222));
#34072=CARTESIAN_POINT('Ctrl Pts',(3.59773203505403,-1.59326849094606,36.0713505983866));
#34073=CARTESIAN_POINT('Ctrl Pts',(3.54719143757431,-1.69880013692002,36.0654255136511));
#34074=CARTESIAN_POINT('Ctrl Pts',(3.49655766018267,-1.80452634785695,36.0594895050464));
#34075=CARTESIAN_POINT('Ctrl Pts',(3.4412518234525,-1.90786443959993,36.0535534964416));
#34076=CARTESIAN_POINT('Ctrl Pts',(3.38154295267334,-2.00839643975617,36.0476174878369));
#34077=CARTESIAN_POINT('Ctrl Pts',(3.32921850769105,-2.09649526062636,36.0424156082569));
#34078=CARTESIAN_POINT('Ctrl Pts',(3.27351353645545,-2.18243944889097,36.0372137286769));
#34079=CARTESIAN_POINT('Ctrl Pts',(3.21463464360123,-2.26596847024816,36.0320118490969));
#34080=CARTESIAN_POINT('Ctrl Pts',(3.14816940685497,-2.36025992021537,36.026139725131));
#34081=CARTESIAN_POINT('Ctrl Pts',(3.07744059861696,-2.45178263820824,36.0202676011652));
#34082=CARTESIAN_POINT('Ctrl Pts',(3.00270672808036,-2.54012623803246,36.0143954771994));
#34083=CARTESIAN_POINT('Ctrl Pts',(2.92806975149084,-2.62835529862533,36.0085309665588));
#34084=CARTESIAN_POINT('Ctrl Pts',(2.84943830341971,-2.71341312508545,36.0026664559183));
#34085=CARTESIAN_POINT('Ctrl Pts',(2.7671139252641,-2.79491851842044,35.9968019452778));
#34086=CARTESIAN_POINT('Ctrl Pts',(2.68487425807463,-2.87634004351652,35.9909434691604));
#34087=CARTESIAN_POINT('Ctrl Pts',(2.59894951117365,-2.95421611717767,35.985084993043));
#34088=CARTESIAN_POINT('Ctrl Pts',(2.50968077474067,-3.02819936742894,35.9792265169256));
#34089=CARTESIAN_POINT('Ctrl Pts',(2.41689205377746,-3.1050998752419,35.9731370333342));
#34090=CARTESIAN_POINT('Ctrl Pts',(2.32049049587995,-3.17779389798758,35.9670475497429));
#34091=CARTESIAN_POINT('Ctrl Pts',(2.22090081590631,-3.24593415920698,35.9609580661516));
#34092=CARTESIAN_POINT('Ctrl Pts',(2.12520019040444,-3.31141349022082,35.9551063816313));
#34093=CARTESIAN_POINT('Ctrl Pts',(2.02655614087375,-3.37268778603635,35.9492546971111));
#34094=CARTESIAN_POINT('Ctrl Pts',(1.92537772850614,-3.42949115796681,35.9434030125909));
#34095=CARTESIAN_POINT('Ctrl Pts',(1.8242147480458,-3.48628586614828,35.9375522205798));
#34096=CARTESIAN_POINT('Ctrl Pts',(1.72051853370941,-3.53861080397351,35.9317014285687));
#34097=CARTESIAN_POINT('Ctrl Pts',(1.61472432391119,-3.58624516141459,35.9258506365576));
#34098=CARTESIAN_POINT('Ctrl Pts',(1.50892062558798,-3.63388379111019,35.9199993197976));
#34099=CARTESIAN_POINT('Ctrl Pts',(1.40101893473241,-3.67683083438635,35.9141480030377));
#34100=CARTESIAN_POINT('Ctrl Pts',(1.29147545916237,-3.71491320738202,35.9082966862778));
#34101=CARTESIAN_POINT('Ctrl Pts',(1.18189562625586,-3.75300821986755,35.9024434274734));
#34102=CARTESIAN_POINT('Ctrl Pts',(1.07067331540675,-3.78623521590995,35.8965901686691));
#34103=CARTESIAN_POINT('Ctrl Pts',(0.958280226486698,-3.81447086861659,
35.8907369098648));
#34104=CARTESIAN_POINT('Ctrl Pts',(0.845759268505086,-3.84273864488571,
35.8848769918369));
#34105=CARTESIAN_POINT('Ctrl Pts',(0.732065275031789,-3.86600364264212,
35.8790170738089));
#34106=CARTESIAN_POINT('Ctrl Pts',(0.617680580600549,-3.88419357143139,
35.873157155781));
#34107=CARTESIAN_POINT('Ctrl Pts',(0.503218867680946,-3.90239574802031,
35.8672932921026));
#34108=CARTESIAN_POINT('Ctrl Pts',(0.388065937513293,-3.91551600466352,
35.8614294284241));
#34109=CARTESIAN_POINT('Ctrl Pts',(0.272707948110416,-3.92353404152907,
35.8555655647457));
#34110=CARTESIAN_POINT('Ctrl Pts',(0.1571797779379,-3.93156390692675,35.8496930504585));
#34111=CARTESIAN_POINT('Ctrl Pts',(0.0414463565074991,-3.93447651968868,
35.8438205361713));
#34112=CARTESIAN_POINT('Ctrl Pts',(-0.0740073703216252,-3.93230363898035,
35.8379480218841));
#34113=CARTESIAN_POINT('Ctrl Pts',(-0.105916305245342,-3.93170310133619,
35.8363249848339));
#34114=CARTESIAN_POINT('Ctrl Pts',(-0.137803915726344,-3.93071441185742,
35.8347019477837));
#34115=CARTESIAN_POINT('Ctrl Pts',(-0.169660074222265,-3.929338934123,35.8330789107334));
#34116=CARTESIAN_POINT('Ctrl Pts',(-0.284915182996696,-3.92436247608846,
35.8272067867675));
#34117=CARTESIAN_POINT('Ctrl Pts',(-0.400144376111135,-3.91430239267515,
35.8213346628015));
#34118=CARTESIAN_POINT('Ctrl Pts',(-0.514862652605059,-3.89915445307729,
35.8154625388356));
#34119=CARTESIAN_POINT('Ctrl Pts',(-0.62943219457563,-3.8840261530839,35.8095980281949));
#34120=CARTESIAN_POINT('Ctrl Pts',(-0.743491731159177,-3.86382316858314,
35.8037335175543));
#34121=CARTESIAN_POINT('Ctrl Pts',(-0.856557568373406,-3.83859324910341,
35.7978690069137));
#34122=CARTESIAN_POINT('Ctrl Pts',(-0.969507061966085,-3.81338929095979,
35.7920105307961));
#34123=CARTESIAN_POINT('Ctrl Pts',(-1.08146448894426,-3.78316877600975,
35.7861520546786));
#34124=CARTESIAN_POINT('Ctrl Pts',(-1.19195324869756,-3.7480310101331,35.7802935785611));
#34125=CARTESIAN_POINT('Ctrl Pts',(-1.30679872660717,-3.71150771560258,
35.7742040949698));
#34126=CARTESIAN_POINT('Ctrl Pts',(-1.4200568803427,-3.66967146433403,35.7681146113785));
#34127=CARTESIAN_POINT('Ctrl Pts',(-1.5312060032593,-3.62269197912032,35.7620251277872));
#34128=CARTESIAN_POINT('Ctrl Pts',(-1.63801466646809,-3.57754707934744,
35.7561734432669));
#34129=CARTESIAN_POINT('Ctrl Pts',(-1.74287550973644,-3.52765327827911,
35.7503217587465));
#34130=CARTESIAN_POINT('Ctrl Pts',(-1.84534376791724,-3.47321110475724,
35.7444700742262));
#34131=CARTESIAN_POINT('Ctrl Pts',(-1.94779639746115,-3.41877723485033,
35.738619282215));
#34132=CARTESIAN_POINT('Ctrl Pts',(-2.0478568025135,-3.35979656575146,35.7327684902038));
#34133=CARTESIAN_POINT('Ctrl Pts',(-2.14510400419289,-3.29651601106314,
35.7269176981926));
#34134=CARTESIAN_POINT('Ctrl Pts',(-2.24235992782914,-3.233229780836,35.7210663814325));
#34135=CARTESIAN_POINT('Ctrl Pts',(-2.33680179998934,-3.16564312387548,
35.7152150646724));
#34136=CARTESIAN_POINT('Ctrl Pts',(-2.42803746981478,-3.09404638704326,
35.7093637479124));
#34137=CARTESIAN_POINT('Ctrl Pts',(-2.51930342063967,-3.02242588734775,
35.703510489108));
#34138=CARTESIAN_POINT('Ctrl Pts',(-2.60736072811292,-2.94679291637804,
35.6976572303035));
#34139=CARTESIAN_POINT('Ctrl Pts',(-2.69185073787341,-2.86747774272276,
35.6918039714991));
#34140=CARTESIAN_POINT('Ctrl Pts',(-2.77643687150012,-2.78807233258669,
35.6859440534711));
#34141=CARTESIAN_POINT('Ctrl Pts',(-2.85744730517025,-2.70497664130493,
35.680084135443));
#34142=CARTESIAN_POINT('Ctrl Pts',(-2.93456058230027,-2.61855746333921,
35.674224217415));
#34143=CARTESIAN_POINT('Ctrl Pts',(-3.01172578200672,-2.53208009686771,
35.6683603537365));
#34144=CARTESIAN_POINT('Ctrl Pts',(-3.08498833944942,-2.44227510737343,
35.6624964900579));
#34145=CARTESIAN_POINT('Ctrl Pts',(-3.15406847912027,-2.34954059956834,
35.6566326263794));
#34146=CARTESIAN_POINT('Ctrl Pts',(-3.22325052860603,-2.25666928606813,
35.6507601120921));
#34147=CARTESIAN_POINT('Ctrl Pts',(-3.28823761480356,-2.16086016971041,
35.6448875978048));
#34148=CARTESIAN_POINT('Ctrl Pts',(-3.34879442180649,-2.06253846521167,
35.6390150835175));
#34149=CARTESIAN_POINT('Ctrl Pts',(-3.36553102499484,-2.0353644539908,35.6373920464683));
#34150=CARTESIAN_POINT('Ctrl Pts',(-3.38192949838553,-2.00799864908361,
35.6357690094191));
#34151=CARTESIAN_POINT('Ctrl Pts',(-3.39798551695636,-1.9804503090345,35.63414597237));
#34152=CARTESIAN_POINT('Ctrl Pts',(-3.45607595395473,-1.88078082341616,
35.6282738484039));
#34153=CARTESIAN_POINT('Ctrl Pts',(-3.50987481252454,-1.77838621886318,
35.6224017244377));
#34154=CARTESIAN_POINT('Ctrl Pts',(-3.55911646351883,-1.67367230935725,
35.6165296004716));
#34155=CARTESIAN_POINT('Ctrl Pts',(-3.60829427173484,-1.56909416351423,
35.6106650898308));
#34156=CARTESIAN_POINT('Ctrl Pts',(-3.65292644795823,-1.46220306325422,
35.60480057919));
#34157=CARTESIAN_POINT('Ctrl Pts',(-3.69279180769145,-1.35343181026859,
35.5989360685492));
#34158=CARTESIAN_POINT('Ctrl Pts',(-3.73261614636621,-1.24477248181989,
35.5930775924314));
#34159=CARTESIAN_POINT('Ctrl Pts',(-3.76768328343449,-1.13423723459942,
35.5872191163137));
#34160=CARTESIAN_POINT('Ctrl Pts',(-3.79781924895605,-1.02228075999645,
35.581360640196));
#34161=CARTESIAN_POINT('Ctrl Pts',(-3.82914351551647,-0.905909693301426,
35.5752711566048));
#34162=CARTESIAN_POINT('Ctrl Pts',(-3.8551395311012,-0.788003423404034,
35.5691816730135));
#34163=CARTESIAN_POINT('Ctrl Pts',(-3.87566820456159,-0.669092645416404,
35.5630921894223));
#34164=CARTESIAN_POINT('Ctrl Pts',(-3.89539521735587,-0.554825425799626,
35.5572405049018));
#34165=CARTESIAN_POINT('Ctrl Pts',(-3.91007380593832,-0.439631125272265,
35.5513888203813));
#34166=CARTESIAN_POINT('Ctrl Pts',(-3.91963237582199,-0.323992343131811,
35.5455371358608));
#34167=CARTESIAN_POINT('Ctrl Pts',(-3.92918948781598,-0.208371198419347,
35.5396863438494));
#34168=CARTESIAN_POINT('Ctrl Pts',(-3.93362809976647,-0.0923061187816158,
35.533835551838));
#34169=CARTESIAN_POINT('Ctrl Pts',(-3.93292850011839,0.0237152473421576,
35.5279847598265));
#34170=CARTESIAN_POINT('Ctrl Pts',(-3.93222883772426,0.139747019249488,
35.5221334430663));
#34171=CARTESIAN_POINT('Ctrl Pts',(-3.92639005011987,0.255734656419345,
35.5162821263061));
#34172=CARTESIAN_POINT('Ctrl Pts',(-3.91544454946725,0.371191298452989,
35.5104308095458));
#34173=CARTESIAN_POINT('Ctrl Pts',(-3.90449541601719,0.486686260396046,
35.5045775507412));
#34174=CARTESIAN_POINT('Ctrl Pts',(-3.88843623829481,0.601649465418135,
35.4987242919365));
#34175=CARTESIAN_POINT('Ctrl Pts',(-3.86735112002908,0.715600666859522,
35.4928710331318));
#34176=CARTESIAN_POINT('Ctrl Pts',(-3.84624201332869,0.829681510018675,
35.4870111151036));
#34177=CARTESIAN_POINT('Ctrl Pts',(-3.82009562839742,0.942747644775464,
35.4811511970754));
#34178=CARTESIAN_POINT('Ctrl Pts',(-3.78904690309602,1.05433038756286,35.4752912790471));
#34179=CARTESIAN_POINT('Ctrl Pts',(-3.75797727179921,1.16598826220463,35.4694274153684));
#34180=CARTESIAN_POINT('Ctrl Pts',(-3.72199885544546,1.27616036402106,35.4635635516896));
#34181=CARTESIAN_POINT('Ctrl Pts',(-3.68129545992388,1.38439616322202,35.4576996880109));
#34182=CARTESIAN_POINT('Ctrl Pts',(-3.64053201710782,1.49279163624931,35.4518271737234));
#34183=CARTESIAN_POINT('Ctrl Pts',(-3.59502984521864,1.59924472687513,35.4459546594359));
#34184=CARTESIAN_POINT('Ctrl Pts',(-3.54501958528189,1.7033276666478,35.4400821451484));
#34185=CARTESIAN_POINT('Ctrl Pts',(-3.53119782161342,1.73209395974999,35.4384591081011));
#34186=CARTESIAN_POINT('Ctrl Pts',(-3.51703196704843,1.76067937158613,35.4368360710538));
#34187=CARTESIAN_POINT('Ctrl Pts',(-3.50252747509735,1.78907526006822,35.4352130340065));
#34188=CARTESIAN_POINT('Ctrl Pts',(-3.45005043833285,1.89181116346021,35.4293409100405));
#34189=CARTESIAN_POINT('Ctrl Pts',(-3.39296142786934,1.99240846515638,35.4234687860746));
#34190=CARTESIAN_POINT('Ctrl Pts',(-3.331458380452,2.09042437302002,35.4175966621086));
#34191=CARTESIAN_POINT('Ctrl Pts',(-3.27003507295682,2.18831320131295,35.4117321514679));
#34192=CARTESIAN_POINT('Ctrl Pts',(-3.20420932695427,2.28362694445509,35.4058676408272));
#34193=CARTESIAN_POINT('Ctrl Pts',(-3.13422580334255,2.37594562514839,35.4000031301866));
#34194=CARTESIAN_POINT('Ctrl Pts',(-3.06431429208025,2.46816931083786,35.394144654069));
#34195=CARTESIAN_POINT('Ctrl Pts',(-2.99025376121517,2.5574037366363,35.3882861779514));
#34196=CARTESIAN_POINT('Ctrl Pts',(-2.91233280283166,2.64325682549969,35.3824277018339));
#34197=CARTESIAN_POINT('Ctrl Pts',(-2.83133931784156,2.73249521538173,35.3763382182426));
#34198=CARTESIAN_POINT('Ctrl Pts',(-2.74617494034244,2.81807973566952,35.3702487346513));
#34199=CARTESIAN_POINT('Ctrl Pts',(-2.65721106180506,2.89960658935326,35.36415925106));
#34200=CARTESIAN_POINT('Ctrl Pts',(-2.57172129192485,2.97794975598523,35.3583075665397));
#34201=CARTESIAN_POINT('Ctrl Pts',(-2.48272353281795,3.05254591346051,35.3524558820193));
#34202=CARTESIAN_POINT('Ctrl Pts',(-2.39058517779383,3.12307404774726,35.346604197499));
#34203=CARTESIAN_POINT('Ctrl Pts',(-2.29846087587175,3.19359142496039,35.3407534054877));
#34204=CARTESIAN_POINT('Ctrl Pts',(-2.20319725864039,3.26004176144352,35.3349026134764));
#34205=CARTESIAN_POINT('Ctrl Pts',(-2.10519400279285,3.32214497134081,35.3290518214652));
#34206=CARTESIAN_POINT('Ctrl Pts',(-2.00718195717924,3.38425375118251,35.3232005047051));
#34207=CARTESIAN_POINT('Ctrl Pts',(-1.90643013371653,3.44201440808012,35.317349187945));
#34208=CARTESIAN_POINT('Ctrl Pts',(-1.80336571094006,3.49519114106877,35.3114978711849));
#34209=CARTESIAN_POINT('Ctrl Pts',(-1.70026708121687,3.54838552334535,35.3056446123805));
#34210=CARTESIAN_POINT('Ctrl Pts',(-1.59485469315812,3.59699276705317,35.2997913535761));
#34211=CARTESIAN_POINT('Ctrl Pts',(-1.48757809164367,3.64082414039209,35.2939380947716));
#34212=CARTESIAN_POINT('Ctrl Pts',(-1.38017944206958,3.68470538046795,35.2880781767436));
#34213=CARTESIAN_POINT('Ctrl Pts',(-1.27091272869601,3.72379974862621,35.2822182587155));
#34214=CARTESIAN_POINT('Ctrl Pts',(-1.16024523484106,3.75796753512169,35.2763583406874));
#34215=CARTESIAN_POINT('Ctrl Pts',(-1.04950322539493,3.79215832776579,35.2704944770088));
#34216=CARTESIAN_POINT('Ctrl Pts',(-0.937358956447254,3.82141582942803,
35.2646306133302));
#34217=CARTESIAN_POINT('Ctrl Pts',(-0.824290841697528,3.84565125931793,
35.2587667496516));
#34218=CARTESIAN_POINT('Ctrl Pts',(-0.711055924294302,3.86992244229369,
35.2528942353643));
#34219=CARTESIAN_POINT('Ctrl Pts',(-0.596894847145015,3.88915669855326,
35.2470217210769));
#34220=CARTESIAN_POINT('Ctrl Pts',(-0.482292178867151,3.90331695538597,
35.2411492067896));
#34221=CARTESIAN_POINT('Ctrl Pts',(-0.450618458309539,3.90723054679429,
35.2395261697408));
#34222=CARTESIAN_POINT('Ctrl Pts',(-0.418911010076204,3.9107568669515,35.237903132692));
#34223=CARTESIAN_POINT('Ctrl Pts',(-0.387180052773377,3.91389583493664,
35.2362800956432));
#34224=CARTESIAN_POINT('Ctrl Pts',(-0.272377919957184,3.92525257454261,
35.2304079716771));
#34225=CARTESIAN_POINT('Ctrl Pts',(-0.156883226493117,3.93157301805287,
35.2245358477111));
#34226=CARTESIAN_POINT('Ctrl Pts',(-0.0411755108716569,3.93278445599355,
35.2186637237451));
#34227=CARTESIAN_POINT('Ctrl Pts',(0.0743821873989408,3.93399432328088,
35.2127992131043));
#34228=CARTESIAN_POINT('Ctrl Pts',(0.190151949021274,3.93010835329838,35.2069347024636));
#34229=CARTESIAN_POINT('Ctrl Pts',(0.305648185573892,3.92110548017461,35.2010701918229));
#34230=CARTESIAN_POINT('Ctrl Pts',(0.421025577648185,3.91211187091772,35.1952117157053));
#34231=CARTESIAN_POINT('Ctrl Pts',(0.536129594798608,3.89801186327134,35.1893532395877));
#34232=CARTESIAN_POINT('Ctrl Pts',(0.650474386927192,3.87883643274007,35.18349476347));
#34233=CARTESIAN_POINT('Ctrl Pts',(0.769327945674279,3.85890488958255,35.1774052798788));
#34234=CARTESIAN_POINT('Ctrl Pts',(0.887360718078619,3.83348942291053,35.1713157962875));
#34235=CARTESIAN_POINT('Ctrl Pts',(1.00403225191212,3.80268434623757,35.1652263126963));
#34236=CARTESIAN_POINT('Ctrl Pts',(1.11614767159814,3.77308223176998,35.1593746281758));
#34237=CARTESIAN_POINT('Ctrl Pts',(1.22700573513248,3.73850366057662,35.1535229436554));
#34238=CARTESIAN_POINT('Ctrl Pts',(1.33613780774355,3.69908431354548,35.147671259135));
#34239=CARTESIAN_POINT('Ctrl Pts',(1.44525323534139,3.65967097882162,35.1418204671237));
#34240=CARTESIAN_POINT('Ctrl Pts',(1.55264280672405,3.61541847668629,35.1359696751124));
#34241=CARTESIAN_POINT('Ctrl Pts',(1.65785488154545,3.56651176806357,35.1301188831011));
#34242=CARTESIAN_POINT('Ctrl Pts',(1.76307639268116,3.51760067307098,35.1242675663409));
#34243=CARTESIAN_POINT('Ctrl Pts',(1.86611964411228,3.46403471605469,35.1184162495808));
#34244=CARTESIAN_POINT('Ctrl Pts',(1.9665553980936,3.40604592837926,35.1125649328206));
#34245=CARTESIAN_POINT('Ctrl Pts',(2.06702448656943,3.34803789430154,35.1067116740162));
#34246=CARTESIAN_POINT('Ctrl Pts',(2.16488399892109,3.2856043172812,35.1008584152117));
#34247=CARTESIAN_POINT('Ctrl Pts',(2.25973221776311,3.21902148237682,35.0950051564072));
#34248=CARTESIAN_POINT('Ctrl Pts',(2.3546883449552,3.15236289651005,35.0891452383791));
#34249=CARTESIAN_POINT('Ctrl Pts',(2.44662600199909,3.08154586825707,35.083285320351));
#34250=CARTESIAN_POINT('Ctrl Pts',(2.53517513579125,3.00688809749645,35.0774254023229));
#34251=CARTESIAN_POINT('Ctrl Pts',(2.62378389224925,2.93218005752225,35.0715615386443));
#34252=CARTESIAN_POINT('Ctrl Pts',(2.70899927913914,2.85362640516566,35.0656976749657));
#34253=CARTESIAN_POINT('Ctrl Pts',(2.79048808283301,2.77158172521883,35.0598338112871));
#34254=CARTESIAN_POINT('Ctrl Pts',(2.87209710210487,2.68941600964288,35.0539612969997));
#34255=CARTESIAN_POINT('Ctrl Pts',(2.94996828894416,2.60374929259215,35.0480887827123));
#34256=CARTESIAN_POINT('Ctrl Pts',(3.02380861326748,2.51496927820786,35.0422162684249));
#34257=CARTESIAN_POINT('Ctrl Pts',(3.04421649585024,2.49043238558377,35.0405932313765));
#34258=CARTESIAN_POINT('Ctrl Pts',(3.06431673688228,2.46565785194012,35.0389701943281));
#34259=CARTESIAN_POINT('Ctrl Pts',(3.08410374667262,2.44065423191403,35.0373471572797));
#34260=CARTESIAN_POINT('Ctrl Pts',(3.15563766634446,2.35026124351392,35.0314795601503));
#34261=CARTESIAN_POINT('Ctrl Pts',(3.2233192179815,2.25656266143007,35.0256119630209));
#34262=CARTESIAN_POINT('Ctrl Pts',(3.2868267905791,2.15992098205734,35.0197443658915));
#34263=CARTESIAN_POINT('Ctrl Pts',(3.35024046023304,2.06342219805599,35.013885444651));
#34264=CARTESIAN_POINT('Ctrl Pts',(3.40949220357858,1.96398931682529,35.0080265234105));
#34265=CARTESIAN_POINT('Ctrl Pts',(3.46430055068524,1.86201790929141,35.00216760217));
#34266=CARTESIAN_POINT('Ctrl Pts',(3.47105962727098,1.84944258838753,35.0014450681133));
#34267=CARTESIAN_POINT('Ctrl Pts',(3.47775117867621,1.83682870064933,35.0007225340567));
#34268=CARTESIAN_POINT('Ctrl Pts',(3.48437472100057,1.8241770209199,35.));
#34269=CARTESIAN_POINT('Origin',(0.,0.,4.68922655072688));
#34270=CARTESIAN_POINT('',(-1.47525540431025,-2.86526422072265,37.4085260041042));
#34271=CARTESIAN_POINT('',(-1.47642197926485,-2.86757701908443,37.6538374878572));
#34272=CARTESIAN_POINT('',(-1.47525540501186,-2.86526422036142,4.68922655072688));
#34273=CARTESIAN_POINT('',(3.0778063018882,-0.968536646922758,38.0000000000001));
#34274=CARTESIAN_POINT('Ctrl Pts',(-1.47642197926477,-2.86757701908447,
37.6538374878573));
#34275=CARTESIAN_POINT('Ctrl Pts',(-0.665155101486716,-3.27567489825073,
37.7100277566941));
#34276=CARTESIAN_POINT('Ctrl Pts',(1.38130508422518,-3.40042127156339,37.8254152607417));
#34277=CARTESIAN_POINT('Ctrl Pts',(2.78385737807687,-1.87794914020384,37.9408027647893));
#34278=CARTESIAN_POINT('Ctrl Pts',(3.0778063018882,-0.968536646922758,38.0000000000001));
#34279=CARTESIAN_POINT('',(1.92911062273198,2.58159829713351,37.9999969413403));
#34280=CARTESIAN_POINT('Origin',(0.,0.,38.));
#34281=CARTESIAN_POINT('',(3.22274953375635,0.00173354353987881,37.8165056021994));
#34282=CARTESIAN_POINT('Ctrl Pts',(3.222749531205,0.00173828016955539,37.8165059165414));
#34283=CARTESIAN_POINT('Ctrl Pts',(3.22270305071438,0.0879125241068303,
37.8222247873387));
#34284=CARTESIAN_POINT('Ctrl Pts',(3.21920019789002,0.174060452734954,37.8278510718186));
#34285=CARTESIAN_POINT('Ctrl Pts',(3.2114797988416,0.269454144514142,37.8339081349421));
#34286=CARTESIAN_POINT('Ctrl Pts',(3.21067053001022,0.278931510071132,37.8345079924864));
#34287=CARTESIAN_POINT('Ctrl Pts',(3.2092464328258,0.294781062059853,37.8355078136478));
#34288=CARTESIAN_POINT('Ctrl Pts',(3.20865456251314,0.301155178058178,37.835908996707));
#34289=CARTESIAN_POINT('Ctrl Pts',(3.20754096814088,0.312771891365883,37.8366384362922));
#34290=CARTESIAN_POINT('Ctrl Pts',(3.2070253751692,0.318015034703768,37.836967029785));
#34291=CARTESIAN_POINT('Ctrl Pts',(3.20593683907471,0.328812599313765,37.8376423829336));
#34292=CARTESIAN_POINT('Ctrl Pts',(3.20536232519363,0.334366724584944,37.8379890372753));
#34293=CARTESIAN_POINT('Ctrl Pts',(3.20402360875131,0.346988193085497,37.8387751375784));
#34294=CARTESIAN_POINT('Ctrl Pts',(3.20325045895787,0.354054502934622,37.8392140737816));
#34295=CARTESIAN_POINT('Ctrl Pts',(3.20118373404302,0.372382545982474,37.8403496410081));
#34296=CARTESIAN_POINT('Ctrl Pts',(3.19985409722441,0.383640228532662,37.8410442892656));
#34297=CARTESIAN_POINT('Ctrl Pts',(3.19108503739539,0.454666263385874,37.8454102006503));
#34298=CARTESIAN_POINT('Ctrl Pts',(3.1820302095878,0.514227520546008,37.8489966822654));
#34299=CARTESIAN_POINT('Ctrl Pts',(3.16366679900411,0.615771813209107,37.8550362213012));
#34300=CARTESIAN_POINT('Ctrl Pts',(3.1551785212053,0.657883962557299,37.8575185671406));
#34301=CARTESIAN_POINT('Ctrl Pts',(3.09705571057058,0.919161018413947,37.8728485623131));
#34302=CARTESIAN_POINT('Ctrl Pts',(3.02545318345635,1.13280770928991,37.8851126266627));
#34303=CARTESIAN_POINT('Ctrl Pts',(2.89150874849534,1.42650354757404,37.9034389615986));
#34304=CARTESIAN_POINT('Ctrl Pts',(2.84676610907895,1.51382154709284,37.9090837800931));
#34305=CARTESIAN_POINT('Ctrl Pts',(2.76897445235689,1.64995383043231,37.9183162286303));
#34306=CARTESIAN_POINT('Ctrl Pts',(2.73844702740723,1.70013951790317,37.9218187002717));
#34307=CARTESIAN_POINT('Ctrl Pts',(2.69709104329107,1.76412079276401,37.9264275422393));
#34308=CARTESIAN_POINT('Ctrl Pts',(2.68749641232533,1.7787032586588,37.927487903642));
#34309=CARTESIAN_POINT('Ctrl Pts',(2.67171291233598,1.80227265496957,37.9292182942922));
#34310=CARTESIAN_POINT('Ctrl Pts',(2.66559595145052,1.81130749122718,37.9298856027177));
#34311=CARTESIAN_POINT('Ctrl Pts',(2.65375232712182,1.82861075903095,37.9311714103812));
#34312=CARTESIAN_POINT('Ctrl Pts',(2.64803259611736,1.83688379817252,37.9317896403862));
#34313=CARTESIAN_POINT('Ctrl Pts',(2.63485785912359,1.85575036666307,37.9332075188928));
#34314=CARTESIAN_POINT('Ctrl Pts',(2.62737755804495,1.86632594172695,37.9340081330577));
#34315=CARTESIAN_POINT('Ctrl Pts',(2.60735435208714,1.89427559330572,37.9361397271336));
#34316=CARTESIAN_POINT('Ctrl Pts',(2.59470173952829,1.91156992752261,37.9374749398502));
#34317=CARTESIAN_POINT('Ctrl Pts',(2.49592050226965,2.04380213864549,37.9478116764587));
#34318=CARTESIAN_POINT('Ctrl Pts',(2.402379485937,2.15297679446978,37.9571075650017));
#34319=CARTESIAN_POINT('Ctrl Pts',(2.18612439940587,2.3736751443618,37.9775951997114));
#34320=CARTESIAN_POINT('Ctrl Pts',(2.06149009590583,2.48267715660793,37.988830446671));
#34321=CARTESIAN_POINT('Ctrl Pts',(1.92911062273198,2.58159829713351,37.9999969413403));
#34322=CARTESIAN_POINT('Ctrl Pts',(-1.47525540431025,-2.86526422072265,
37.4085260041042));
#34323=CARTESIAN_POINT('Ctrl Pts',(-1.43625760423782,-2.88534324690704,
37.4114783217196));
#34324=CARTESIAN_POINT('Ctrl Pts',(-1.39683575020098,-2.90463337997842,
37.4144193805815));
#34325=CARTESIAN_POINT('Ctrl Pts',(-1.27393816816533,-2.96168666266681,
37.4234325092417));
#34326=CARTESIAN_POINT('Ctrl Pts',(-1.1892482247323,-2.9966979124969,37.429427020127));
#34327=CARTESIAN_POINT('Ctrl Pts',(-1.09009691860782,-3.03282046492186,
37.4361111154649));
#34328=CARTESIAN_POINT('Ctrl Pts',(-1.0769890306239,-3.03749994383052,37.4369881523242));
#34329=CARTESIAN_POINT('Ctrl Pts',(-1.05717493303045,-3.04442913262363,
37.4383035141713));
#34330=CARTESIAN_POINT('Ctrl Pts',(-1.05049115905415,-3.04674185148841,
37.4387454441221));
#34331=CARTESIAN_POINT('Ctrl Pts',(-1.03851967456026,-3.05084014569193,
37.4395337580483));
#34332=CARTESIAN_POINT('Ctrl Pts',(-1.03323490810244,-3.05263399955876,
37.4398806263606));
#34333=CARTESIAN_POINT('Ctrl Pts',(-1.02177956153736,-3.05648923004023,
37.4406300496742));
#34334=CARTESIAN_POINT('Ctrl Pts',(-1.01560741011654,-3.0585456472008,37.4410323099559));
#34335=CARTESIAN_POINT('Ctrl Pts',(-0.998341982499454,-3.06424005945056,
37.4421533973977));
#34336=CARTESIAN_POINT('Ctrl Pts',(-0.987234969882515,-3.0678365308348,
37.4428698150333));
#34337=CARTESIAN_POINT('Ctrl Pts',(-0.92237377082824,-3.08844997402597,
37.4470269220475));
#34338=CARTESIAN_POINT('Ctrl Pts',(-0.868196327896372,-3.10411543744507,
37.4503933551825));
#34339=CARTESIAN_POINT('Ctrl Pts',(-0.567968942834488,-3.18244995353801,
37.4686115598272));
#34340=CARTESIAN_POINT('Ctrl Pts',(-0.315569757793848,-3.21730000377383,
37.4823896948693));
#34341=CARTESIAN_POINT('Ctrl Pts',(0.102172048858668,-3.22529598914287,
37.505990032542));
#34342=CARTESIAN_POINT('Ctrl Pts',(0.265998739668756,-3.21593028080837,
37.5154334030571));
#34343=CARTESIAN_POINT('Ctrl Pts',(0.450099879470417,-3.19123917122849,
37.5266056965123));
#34344=CARTESIAN_POINT('Ctrl Pts',(0.47177886739132,-3.18810633660193,37.5279298974547));
#34345=CARTESIAN_POINT('Ctrl Pts',(0.506362463765492,-3.1827481905488,37.530056797019));
#34346=CARTESIAN_POINT('Ctrl Pts',(0.519288604395263,-3.18066476173729,
37.5308549945278));
#34347=CARTESIAN_POINT('Ctrl Pts',(0.542142228265927,-3.17683820086012,
37.5322720981139));
#34348=CARTESIAN_POINT('Ctrl Pts',(0.552074959888118,-3.17512714471595,
37.5328899751805));
#34349=CARTESIAN_POINT('Ctrl Pts',(0.572681199104011,-3.17147780788289,
37.534175972722));
#34350=CARTESIAN_POINT('Ctrl Pts',(0.58335325957357,-3.16953217551716,37.5348443208466));
#34351=CARTESIAN_POINT('Ctrl Pts',(0.610891962848549,-3.16436777485636,
37.5365750642616));
#34352=CARTESIAN_POINT('Ctrl Pts',(0.627742901766128,-3.16106805300211,
37.5376400362361));
#34353=CARTESIAN_POINT('Ctrl Pts',(0.699516743483176,-3.14641689040722,
37.5422019819395));
#34354=CARTESIAN_POINT('Ctrl Pts',(0.754161905297265,-3.1337680363353,37.5457402667464));
#34355=CARTESIAN_POINT('Ctrl Pts',(0.897409856562916,-3.09664642239335,
37.555194229315));
#34356=CARTESIAN_POINT('Ctrl Pts',(0.98533890770676,-3.06979937999765,37.5611815026519));
#34357=CARTESIAN_POINT('Ctrl Pts',(1.2095339777098,-2.99072159863251,37.5769081150617));
#34358=CARTESIAN_POINT('Ctrl Pts',(1.34361342306006,-2.93293127891763,37.5867751799219));
#34359=CARTESIAN_POINT('Ctrl Pts',(1.64055446299926,-2.78029852200403,37.6093749174947));
#34360=CARTESIAN_POINT('Ctrl Pts',(1.79997494065692,-2.67984805879226,37.6220741106077));
#34361=CARTESIAN_POINT('Ctrl Pts',(1.9613994561847,-2.55719460177184,37.6349237909817));
#34362=CARTESIAN_POINT('Ctrl Pts',(1.97300052435852,-2.54825450221348,37.6358470784723));
#34363=CARTESIAN_POINT('Ctrl Pts',(1.99015393674327,-2.53484824568232,37.6372114851217));
#34364=CARTESIAN_POINT('Ctrl Pts',(1.99575287536791,-2.53044240862144,37.637656708983));
#34365=CARTESIAN_POINT('Ctrl Pts',(2.00571489348871,-2.5225496074878,37.6384485903369));
#34366=CARTESIAN_POINT('Ctrl Pts',(2.01008355105668,-2.51906984333524,37.6387957505675));
#34367=CARTESIAN_POINT('Ctrl Pts',(2.01446052691476,-2.51556481699289,37.6391434612459));
#34368=CARTESIAN_POINT('Ctrl Pts',(2.01447780796669,-2.51555097825504,37.6391448340657));
#34369=CARTESIAN_POINT('Ctrl Pts',(2.01451209387071,-2.51552352138144,37.6391475577606));
#34370=CARTESIAN_POINT('Ctrl Pts',(2.01452909869127,-2.5155099032802,37.6391489086332));
#34371=CARTESIAN_POINT('Ctrl Pts',(2.0145628373658,-2.51548288351646,37.6391515888495));
#34372=CARTESIAN_POINT('Ctrl Pts',(2.01457957132563,-2.51546948177812,37.6391529182017));
#34373=CARTESIAN_POINT('Ctrl Pts',(2.01461277389525,-2.51544289026868,37.6391555558235));
#34374=CARTESIAN_POINT('Ctrl Pts',(2.01462924241462,-2.51542970057863,37.639156864086));
#34375=CARTESIAN_POINT('Ctrl Pts',(2.0146619193043,-2.51540352902598,37.6391594599418));
#34376=CARTESIAN_POINT('Ctrl Pts',(2.01467812761216,-2.51539054722172,37.6391607475302));
#34377=CARTESIAN_POINT('Ctrl Pts',(2.01471028907978,-2.51536478746003,37.6391633024351));
#34378=CARTESIAN_POINT('Ctrl Pts',(2.01472624225204,-2.51535200950061,37.6391645697527));
#34379=CARTESIAN_POINT('Ctrl Pts',(2.01972807099056,-2.51134563322859,37.6395619138407));
#34380=CARTESIAN_POINT('Ctrl Pts',(2.02470211271556,-2.50733717850673,37.6399569153863));
#34381=CARTESIAN_POINT('Ctrl Pts',(2.03827249452963,-2.49633443583687,37.6410343068212));
#34382=CARTESIAN_POINT('Ctrl Pts',(2.04684482313504,-2.48931047799182,37.6417145931564));
#34383=CARTESIAN_POINT('Ctrl Pts',(2.06606395237776,-2.47339638665036,37.6432395665484));
#34384=CARTESIAN_POINT('Ctrl Pts',(2.07669000471623,-2.4644814019076,37.6440825502383));
#34385=CARTESIAN_POINT('Ctrl Pts',(2.10951810837679,-2.43657637541224,37.6466875629647));
#34386=CARTESIAN_POINT('Ctrl Pts',(2.13152033616147,-2.41735232524608,37.6484345170127));
#34387=CARTESIAN_POINT('Ctrl Pts',(2.21662868366218,-2.34092479432583,37.6552100180404));
#34388=CARTESIAN_POINT('Ctrl Pts',(2.277722411028,-2.28152455949615,37.6601136487935));
#34389=CARTESIAN_POINT('Ctrl Pts',(2.47910493352838,-2.06956152673026,37.6767133184336));
#34390=CARTESIAN_POINT('Ctrl Pts',(2.60699792545665,-1.90594121404209,37.6880679711775));
#34391=CARTESIAN_POINT('Ctrl Pts',(2.79364918059233,-1.61285988383586,37.7078258502478));
#34392=CARTESIAN_POINT('Ctrl Pts',(2.86118440054439,-1.48976823541654,37.7159683100511));
#34393=CARTESIAN_POINT('Ctrl Pts',(2.92950456987935,-1.3433449777783,37.7256914787533));
#34394=CARTESIAN_POINT('Ctrl Pts',(2.93833337958235,-1.32392207894861,37.7269817553788));
#34395=CARTESIAN_POINT('Ctrl Pts',(2.95220046439086,-1.29259315699834,37.7290644168006));
#34396=CARTESIAN_POINT('Ctrl Pts',(2.9573611778658,-1.28074178017141,37.7298525949595));
#34397=CARTESIAN_POINT('Ctrl Pts',(2.96640875182672,-1.25961809982176,37.7312581549325));
#34398=CARTESIAN_POINT('Ctrl Pts',(2.97032380494049,-1.25035800092514,37.7318745637));
#34399=CARTESIAN_POINT('Ctrl Pts',(2.97840216178564,-1.23099855951164,37.7331638276924));
#34400=CARTESIAN_POINT('Ctrl Pts',(2.98255756835005,-1.22089607977979,37.7338369421164));
#34401=CARTESIAN_POINT('Ctrl Pts',(2.99324152136314,-1.19454154661972,37.7355938605544));
#34402=CARTESIAN_POINT('Ctrl Pts',(2.9996890194264,-1.17825722107829,37.7366803906561));
#34403=CARTESIAN_POINT('Ctrl Pts',(3.02738045597171,-1.10661678915694,37.7414651034141));
#34404=CARTESIAN_POINT('Ctrl Pts',(3.04722600175411,-1.05073597301318,37.745209778755));
#34405=CARTESIAN_POINT('Ctrl Pts',(3.09618601212435,-0.899794217254751,
37.7553646995311));
#34406=CARTESIAN_POINT('Ctrl Pts',(3.12246079401988,-0.803886135467158,
37.7618604483947));
#34407=CARTESIAN_POINT('Ctrl Pts',(3.19655906508416,-0.474311713053508,
37.7842838470966));
#34408=CARTESIAN_POINT('Ctrl Pts',(3.22287775861272,-0.236643276283802,
37.8006859445876));
#34409=CARTESIAN_POINT('Ctrl Pts',(3.22274953375635,0.00173354353987881,
37.8165056021994));
#34410=CARTESIAN_POINT('Origin',(0.,0.,4.68922655072688));
#34411=CARTESIAN_POINT('',(-1.47525533429856,-2.86526425676998,36.1542047394732));
#34412=CARTESIAN_POINT('',(-1.47525545662511,-2.865264193787,36.4017031386693));
#34413=CARTESIAN_POINT('',(-1.47525540501186,-2.86526422036142,4.68922655072688));
#34414=CARTESIAN_POINT('',(3.22710931890567,0.00161487490920624,36.8107734492731));
#34415=CARTESIAN_POINT('Ctrl Pts',(3.22274952067548,0.00175769336351857,
36.8082682062519));
#34416=CARTESIAN_POINT('Ctrl Pts',(3.22276605484594,-0.0285578844381251,
36.80650283569));
#34417=CARTESIAN_POINT('Ctrl Pts',(3.22235483219543,-0.05887312616645,36.8047522247304));
#34418=CARTESIAN_POINT('Ctrl Pts',(3.21327137318411,-0.387005561556071,
36.7859214086916));
#34419=CARTESIAN_POINT('Ctrl Pts',(3.16376992247395,-0.68224905193963,36.7698842931772));
#34420=CARTESIAN_POINT('Ctrl Pts',(3.04938585646319,-1.04609995332455,36.7476979918744));
#34421=CARTESIAN_POINT('Ctrl Pts',(3.02128342954484,-1.1246883395346,36.742763256182));
#34422=CARTESIAN_POINT('Ctrl Pts',(2.98285032186027,-1.22028936190716,36.7365420512188));
#34423=CARTESIAN_POINT('Ctrl Pts',(2.9753694133729,-1.23841794118675,36.7353524918587));
#34424=CARTESIAN_POINT('Ctrl Pts',(2.96328290429647,-1.266965558166,36.7334631611481));
#34425=CARTESIAN_POINT('Ctrl Pts',(2.95878664247503,-1.27743058344845,36.7327671204464));
#34426=CARTESIAN_POINT('Ctrl Pts',(2.95025209269912,-1.2970078992249,36.7314584368492));
#34427=CARTESIAN_POINT('Ctrl Pts',(2.94622681528071,-1.30612574068935,36.7308462461957));
#34428=CARTESIAN_POINT('Ctrl Pts',(2.93712178009111,-1.32649371637484,36.7294725934711));
#34429=CARTESIAN_POINT('Ctrl Pts',(2.93201957254121,-1.33773358711513,36.7287103643352));
#34430=CARTESIAN_POINT('Ctrl Pts',(2.91892192023341,-1.36615204620692,36.7267723867528));
#34431=CARTESIAN_POINT('Ctrl Pts',(2.91083939729689,-1.38328976290622,36.7255936367331));
#34432=CARTESIAN_POINT('Ctrl Pts',(2.86351639764259,-1.48137920989517,36.7187880237311));
#34433=CARTESIAN_POINT('Ctrl Pts',(2.82105450547159,-1.56072400536159,36.7130492195396));
#34434=CARTESIAN_POINT('Ctrl Pts',(2.63326649012482,-1.87886563895286,36.6890430908086));
#34435=CARTESIAN_POINT('Ctrl Pts',(2.46050134454939,-2.10002863479042,36.669822646677));
#34436=CARTESIAN_POINT('Ctrl Pts',(2.20945924073325,-2.34728117032595,36.6462732745994));
#34437=CARTESIAN_POINT('Ctrl Pts',(2.1557594856927,-2.39669386755196,36.6414506258617));
#34438=CARTESIAN_POINT('Ctrl Pts',(2.0804396760161,-2.46141884193578,36.6350203875209));
#34439=CARTESIAN_POINT('Ctrl Pts',(2.0602432364287,-2.47834821289421,36.6333272889481));
#34440=CARTESIAN_POINT('Ctrl Pts',(2.02986562523331,-2.50318379611761,36.6308294108307));
#34441=CARTESIAN_POINT('Ctrl Pts',(2.01984151149068,-2.51127932629666,36.6300128964112));
#34442=CARTESIAN_POINT('Ctrl Pts',(2.00160723725369,-2.52582561469292,36.6285419920877));
#34443=CARTESIAN_POINT('Ctrl Pts',(1.99341382175586,-2.5322969633083,36.6278862401827));
#34444=CARTESIAN_POINT('Ctrl Pts',(1.98027247466594,-2.54257299615543,36.6268429385855));
#34445=CARTESIAN_POINT('Ctrl Pts',(1.97534477213949,-2.54640325703751,36.62645360774));
#34446=CARTESIAN_POINT('Ctrl Pts',(1.96619282674201,-2.5534744324519,36.6257340567563));
#34447=CARTESIAN_POINT('Ctrl Pts',(1.96197172778946,-2.55671915723209,36.6254035717015));
#34448=CARTESIAN_POINT('Ctrl Pts',(1.95207787242992,-2.56428555302981,36.624632163286));
#34449=CARTESIAN_POINT('Ctrl Pts',(1.94639880479212,-2.56859886173743,36.624191832511));
#34450=CARTESIAN_POINT('Ctrl Pts',(1.92899148777409,-2.58172901126351,36.6228494776079));
#34451=CARTESIAN_POINT('Ctrl Pts',(1.91721711122963,-2.59048478375062,36.6219516327591));
#34452=CARTESIAN_POINT('Ctrl Pts',(1.75489781846419,-2.70947723984751,36.6097061108786));
#34453=CARTESIAN_POINT('Ctrl Pts',(1.59509190662659,-2.80653453996464,36.5991877727189));
#34454=CARTESIAN_POINT('Ctrl Pts',(1.2958759370638,-2.95439752107189,36.5805075949685));
#34455=CARTESIAN_POINT('Ctrl Pts',(1.15968358011756,-3.01046368765049,36.5723406741485));
#34456=CARTESIAN_POINT('Ctrl Pts',(0.932892404282599,-3.08614478306714,
36.5587297343269));
#34457=CARTESIAN_POINT('Ctrl Pts',(0.844441674176579,-3.111509952806,36.5534208244709));
#34458=CARTESIAN_POINT('Ctrl Pts',(0.700471980442569,-3.14620505278839,
36.5446884902619));
#34459=CARTESIAN_POINT('Ctrl Pts',(0.645580608867946,-3.15792532051728,
36.5413386643411));
#34460=CARTESIAN_POINT('Ctrl Pts',(0.573525407193728,-3.17135322634818,
36.536903343233));
#34461=CARTESIAN_POINT('Ctrl Pts',(0.556612567602607,-3.17436530833754,
36.5358595874755));
#34462=CARTESIAN_POINT('Ctrl Pts',(0.52897770913344,-3.17905928174248,36.5341494268078));
#34463=CARTESIAN_POINT('Ctrl Pts',(0.518269707133551,-3.18082250993434,
36.5334856213996));
#34464=CARTESIAN_POINT('Ctrl Pts',(0.497596464884699,-3.18411949787508,
36.5322017561688));
#34465=CARTESIAN_POINT('Ctrl Pts',(0.487632518424355,-3.18566064449777,
36.5315819396622));
#34466=CARTESIAN_POINT('Ctrl Pts',(0.464709565415272,-3.18909612670047,
36.5301535621975));
#34467=CARTESIAN_POINT('Ctrl Pts',(0.451745981609123,-3.19095826445369,
36.5293439885043));
#34468=CARTESIAN_POINT('Ctrl Pts',(0.417066885607546,-3.19572413789937,
36.5271733542962));
#34469=CARTESIAN_POINT('Ctrl Pts',(0.395332806374885,-3.19848549887924,
36.5258078129339));
#34470=CARTESIAN_POINT('Ctrl Pts',(0.210804253310464,-3.2200207344675,36.5141683524406));
#34471=CARTESIAN_POINT('Ctrl Pts',(0.0468498156986263,-3.22657130235436,
36.5035071245191));
#34472=CARTESIAN_POINT('Ctrl Pts',(-0.370926724992662,-3.21141096296261,
36.4756243991621));
#34473=CARTESIAN_POINT('Ctrl Pts',(-0.622986109466305,-3.17216495732823,
36.4580755360971));
#34474=CARTESIAN_POINT('Ctrl Pts',(-0.921844436026495,-3.08860298168915,
36.4377768145144));
#34475=CARTESIAN_POINT('Ctrl Pts',(-0.975479136866018,-3.07208510679403,
36.4341589201158));
#34476=CARTESIAN_POINT('Ctrl Pts',(-1.03970943635549,-3.05045206800001,
36.4298790289116));
#34477=CARTESIAN_POINT('Ctrl Pts',(-1.05073997555764,-3.04667015687418,
36.4291459310195));
#34478=CARTESIAN_POINT('Ctrl Pts',(-1.06789081565318,-3.04068562500645,
36.4280093161713));
#34479=CARTESIAN_POINT('Ctrl Pts',(-1.07402525303346,-3.03852425066817,
36.4276034256032));
#34480=CARTESIAN_POINT('Ctrl Pts',(-1.0854135811211,-3.03447295164859,36.4268511698193));
#34481=CARTESIAN_POINT('Ctrl Pts',(-1.09066905278063,-3.03258796317373,
36.4265045275812));
#34482=CARTESIAN_POINT('Ctrl Pts',(-1.10257831092685,-3.02828148707774,
36.425720142159));
#34483=CARTESIAN_POINT('Ctrl Pts',(-1.10922901640343,-3.02585172937019,
36.4252828985485));
#34484=CARTESIAN_POINT('Ctrl Pts',(-1.12895768572347,-3.01857030311774,
36.4239880705158));
#34485=CARTESIAN_POINT('Ctrl Pts',(-1.14201241672374,-3.01365555221201,
36.4231341595343));
#34486=CARTESIAN_POINT('Ctrl Pts',(-1.24129942132,-2.9755388743415,36.4166589295455));
#34487=CARTESIAN_POINT('Ctrl Pts',(-1.32610848080994,-2.93872346122117,
36.4112379686349));
#34488=CARTESIAN_POINT('Ctrl Pts',(-1.4313674177628,-2.8875441186618,36.4045101853076));
#34489=CARTESIAN_POINT('Ctrl Pts',(-1.45337870525942,-2.87652800565308,
36.4031033493262));
#34490=CARTESIAN_POINT('Ctrl Pts',(-1.47525545662511,-2.865264193787,36.4017031386693));
#34491=CARTESIAN_POINT('Ctrl Pts',(3.22710931890567,0.00161487490920624,
36.8107734492731));
#34492=CARTESIAN_POINT('Ctrl Pts',(3.22766820945557,0.092902302212634,36.8164301670323));
#34493=CARTESIAN_POINT('Ctrl Pts',(3.18268013141034,1.25374923679401,36.8883978642459));
#34494=CARTESIAN_POINT('Ctrl Pts',(1.77912732379145,3.37157490318388,37.0266765409141));
#34495=CARTESIAN_POINT('Ctrl Pts',(-1.875636683147,3.31885498005365,37.2256094792775));
#34496=CARTESIAN_POINT('Ctrl Pts',(-3.806119388409,0.2150966389413,37.4245424176409));
#34497=CARTESIAN_POINT('Ctrl Pts',(-2.68065523389285,-2.15386545564773,
37.5672850871675));
#34498=CARTESIAN_POINT('Ctrl Pts',(-1.62254331795257,-2.79407246706486,
37.6437167772396));
#34499=CARTESIAN_POINT('Ctrl Pts',(-1.47642197926477,-2.86757701908447,
37.6538374878573));
#34500=CARTESIAN_POINT('Ctrl Pts',(-1.47525533429857,-2.86526425676998,
36.1542047394732));
#34501=CARTESIAN_POINT('Ctrl Pts',(-1.35648519049259,-2.92641613405012,
36.1626885432144));
#34502=CARTESIAN_POINT('Ctrl Pts',(-1.23401696002696,-2.98012972438504,
36.171426215797));
#34503=CARTESIAN_POINT('Ctrl Pts',(-0.871056753745843,-3.11309363011468,
36.1972043428991));
#34504=CARTESIAN_POINT('Ctrl Pts',(-0.62415665607532,-3.17183152281709,
36.2146603565864));
#34505=CARTESIAN_POINT('Ctrl Pts',(-0.315582863209829,-3.20778098899618,
36.2349996513337));
#34506=CARTESIAN_POINT('Ctrl Pts',(-0.258057652374377,-3.21292057905945,
36.2387254237883));
#34507=CARTESIAN_POINT('Ctrl Pts',(-0.188689003787312,-3.21724295097161,
36.2431149691367));
#34508=CARTESIAN_POINT('Ctrl Pts',(-0.176952494959484,-3.21790981388537,
36.2438540833031));
#34509=CARTESIAN_POINT('Ctrl Pts',(-0.158697769992497,-3.21884686376737,
36.2449978860274));
#34510=CARTESIAN_POINT('Ctrl Pts',(-0.152182082262523,-3.21916149489491,
36.2454049970216));
#34511=CARTESIAN_POINT('Ctrl Pts',(-0.140091921436821,-3.21970851840367,
36.2461582237465));
#34512=CARTESIAN_POINT('Ctrl Pts',(-0.134517851565134,-3.21994621667609,
36.246504624429));
#34513=CARTESIAN_POINT('Ctrl Pts',(-0.121899983884943,-3.22045146537396,
36.2472868186752));
#34514=CARTESIAN_POINT('Ctrl Pts',(-0.114855926478386,-3.22071038208709,
36.2477221232154));
#34515=CARTESIAN_POINT('Ctrl Pts',(-0.0940122937803075,-3.2214080568381,
36.2490063209519));
#34516=CARTESIAN_POINT('Ctrl Pts',(-0.0802104780147182,-3.2217812581072,
36.249851628328));
#34517=CARTESIAN_POINT('Ctrl Pts',(0.0221298499941792,-3.22389048050423,
36.2560850492217));
#34518=CARTESIAN_POINT('Ctrl Pts',(0.110712612917276,-3.22206538514645,
36.2612892835029));
#34519=CARTESIAN_POINT('Ctrl Pts',(0.445915510658712,-3.2013154222992,36.2806307746532));
#34520=CARTESIAN_POINT('Ctrl Pts',(0.690145716217482,-3.15768500635991,
36.2940591626006));
#34521=CARTESIAN_POINT('Ctrl Pts',(1.01452756133985,-3.06026212167359,36.3133462070023));
#34522=CARTESIAN_POINT('Ctrl Pts',(1.10089540739617,-3.03026365611643,36.3186227453361));
#34523=CARTESIAN_POINT('Ctrl Pts',(1.23781003456563,-2.97608206240529,36.327306455389));
#34524=CARTESIAN_POINT('Ctrl Pts',(1.28920685994301,-2.95418063542867,36.3306410855843));
#34525=CARTESIAN_POINT('Ctrl Pts',(1.35560046236527,-2.92382608149794,36.3350588579925));
#34526=CARTESIAN_POINT('Ctrl Pts',(1.37113718712766,-2.91657236577657,36.3361006719362));
#34527=CARTESIAN_POINT('Ctrl Pts',(1.39640277016724,-2.90452998414118,36.337808298884));
#34528=CARTESIAN_POINT('Ctrl Pts',(1.40616678114284,-2.89981552936949,36.3384715255641));
#34529=CARTESIAN_POINT('Ctrl Pts',(1.42496266930354,-2.89062287066295,36.3397547264029));
#34530=CARTESIAN_POINT('Ctrl Pts',(1.43399770170545,-2.88615137806843,36.3403744598718));
#34531=CARTESIAN_POINT('Ctrl Pts',(1.45472976009375,-2.87576957325743,36.341803297677));
#34532=CARTESIAN_POINT('Ctrl Pts',(1.46641195118515,-2.86983018568026,36.342613418507));
#34533=CARTESIAN_POINT('Ctrl Pts',(1.49755967260083,-2.85375441088964,36.3447869664951));
#34534=CARTESIAN_POINT('Ctrl Pts',(1.51695816490364,-2.84349030209702,36.3461548952742));
#34535=CARTESIAN_POINT('Ctrl Pts',(1.68083909316897,-2.75462355953177,36.357835068579));
#34536=CARTESIAN_POINT('Ctrl Pts',(1.81919097537173,-2.66527678924624,36.3685375908901));
#34537=CARTESIAN_POINT('Ctrl Pts',(2.15338260351415,-2.41127628278103,36.3965392768757));
#34538=CARTESIAN_POINT('Ctrl Pts',(2.33757028432234,-2.23317501815466,36.4141675774876));
#34539=CARTESIAN_POINT('Ctrl Pts',(2.53323312048606,-1.99294232868106,36.4344160582179));
#34540=CARTESIAN_POINT('Ctrl Pts',(2.56658298813822,-1.94980557244468,36.4379287022976));
#34541=CARTESIAN_POINT('Ctrl Pts',(2.60566044690566,-1.89651913145639,36.4421009236364));
#34542=CARTESIAN_POINT('Ctrl Pts',(2.61244621916695,-1.88716081510612,36.4428275825417));
#34543=CARTESIAN_POINT('Ctrl Pts',(2.62295753273703,-1.87249922315853,36.4439563210097));
#34544=CARTESIAN_POINT('Ctrl Pts',(2.62671759778278,-1.86722098920448,36.4443607233275));
#34545=CARTESIAN_POINT('Ctrl Pts',(2.63368774521397,-1.85737384537279,36.4451115070263));
#34546=CARTESIAN_POINT('Ctrl Pts',(2.63690184234078,-1.85280798122805,36.4454581572087));
#34547=CARTESIAN_POINT('Ctrl Pts',(2.64418024368227,-1.84241116954627,36.4462441981131));
#34548=CARTESIAN_POINT('Ctrl Pts',(2.64823712627546,-1.83657512888788,36.4466830793902));
#34549=CARTESIAN_POINT('Ctrl Pts',(2.65871239544762,-1.82139902013144,36.447818410412));
#34550=CARTESIAN_POINT('Ctrl Pts',(2.66510094696543,-1.81203833942282,36.4485128787553));
#34551=CARTESIAN_POINT('Ctrl Pts',(2.70510337492795,-1.75275647877739,36.4528757988539));
#34552=CARTESIAN_POINT('Ctrl Pts',(2.73736513833007,-1.70193205234039,36.4564596009306));
#34553=CARTESIAN_POINT('Ctrl Pts',(2.93892976009823,-1.36381649689437,36.4794989374551));
#34554=CARTESIAN_POINT('Ctrl Pts',(3.06420210421427,-1.05262467792409,36.4972114672141));
#34555=CARTESIAN_POINT('Ctrl Pts',(3.15914205093584,-0.643036144895613,
36.521630007708));
#34556=CARTESIAN_POINT('Ctrl Pts',(3.17533518873855,-0.557600584126361,
36.526765492885));
#34557=CARTESIAN_POINT('Ctrl Pts',(3.19095975778362,-0.451981742642096,
36.533210627656));
#34558=CARTESIAN_POINT('Ctrl Pts',(3.19368337042743,-0.43231721414448,36.5344146060057));
#34559=CARTESIAN_POINT('Ctrl Pts',(3.19768988748429,-0.401282733161163,
36.5363215020611));
#34560=CARTESIAN_POINT('Ctrl Pts',(3.19909424851081,-0.389928752815022,
36.5370205673367));
#34561=CARTESIAN_POINT('Ctrl Pts',(3.20160785947631,-0.368678505116161,
36.5383317097633));
#34562=CARTESIAN_POINT('Ctrl Pts',(3.20273175667167,-0.358784081663207,
36.5389433152643));
#34563=CARTESIAN_POINT('Ctrl Pts',(3.2051375239809,-0.336691909387495,36.5403114660003));
#34564=CARTESIAN_POINT('Ctrl Pts',(3.20639565045291,-0.324491780416018,
36.5410687525325));
#34565=CARTESIAN_POINT('Ctrl Pts',(3.20939615766952,-0.293672553523231,
36.5429862892245));
#34566=CARTESIAN_POINT('Ctrl Pts',(3.21104615788522,-0.275045112098162,
36.5441494336786));
#34567=CARTESIAN_POINT('Ctrl Pts',(3.21939660122333,-0.170421113847801,
36.5507066252172));
#34568=CARTESIAN_POINT('Ctrl Pts',(3.2228039392682,-0.0842040481459283,
36.5562032879677));
#34569=CARTESIAN_POINT('Ctrl Pts',(3.22263357550004,0.184970274485804,36.5736660170257));
#34570=CARTESIAN_POINT('Ctrl Pts',(3.20694277966631,0.367538399943799,36.5859673833119));
#34571=CARTESIAN_POINT('Ctrl Pts',(3.15894344069144,0.645829823717705,36.6050828408999));
#34572=CARTESIAN_POINT('Ctrl Pts',(3.13749662835673,0.743058334153712,36.6118258198534));
#34573=CARTESIAN_POINT('Ctrl Pts',(3.10457565432211,0.865131329287124,36.620278234588));
#34574=CARTESIAN_POINT('Ctrl Pts',(3.09724088761861,0.89103375506053,36.6220708041795));
#34575=CARTESIAN_POINT('Ctrl Pts',(3.06654473160006,0.994473963037814,36.6292184191876));
#34576=CARTESIAN_POINT('Ctrl Pts',(3.04058708029015,1.07121786073489,36.6344970946243));
#34577=CARTESIAN_POINT('Ctrl Pts',(3.00695581531393,1.15953299579155,36.6404799419706));
#34578=CARTESIAN_POINT('Ctrl Pts',(3.00206897881807,1.17212708571676,36.6413308873444));
#34579=CARTESIAN_POINT('Ctrl Pts',(2.99453543051912,1.19118592291648,36.6426148360029));
#34580=CARTESIAN_POINT('Ctrl Pts',(2.99194672477672,1.19767322165597,36.6430511985206));
#34581=CARTESIAN_POINT('Ctrl Pts',(2.9872538715903,1.20932334375856,36.6438335579084));
#34582=CARTESIAN_POINT('Ctrl Pts',(2.98515741117633,1.21448914159256,36.6441800079051));
#34583=CARTESIAN_POINT('Ctrl Pts',(2.98056009655472,1.22573336116057,36.6449331118216));
#34584=CARTESIAN_POINT('Ctrl Pts',(2.9780540571047,1.23180956183125,36.6453394461138));
#34585=CARTESIAN_POINT('Ctrl Pts',(2.97092667178849,1.24894189853023,36.6464834692871));
#34586=CARTESIAN_POINT('Ctrl Pts',(2.96626216830768,1.2599801246071,36.6472185866358));
#34587=CARTESIAN_POINT('Ctrl Pts',(2.93716503604649,1.32777928414764,36.651723219759));
#34588=CARTESIAN_POINT('Ctrl Pts',(2.91116378962115,1.38385794959682,36.6554032242125));
#34589=CARTESIAN_POINT('Ctrl Pts',(2.76347261567103,1.67977881225645,36.6747539223773));
#34590=CARTESIAN_POINT('Ctrl Pts',(2.61372736611706,1.90444108728551,36.6892804506745));
#34591=CARTESIAN_POINT('Ctrl Pts',(2.34376095287608,2.21665787511883,36.7127248839091));
#34592=CARTESIAN_POINT('Ctrl Pts',(2.24256419857794,2.31898376879698,36.7210616337054));
#34593=CARTESIAN_POINT('Ctrl Pts',(2.11882836152967,2.4284034428552,36.731000513484));
#34594=CARTESIAN_POINT('Ctrl Pts',(2.10263219673709,2.44244032027682,36.7322965821504));
#34595=CARTESIAN_POINT('Ctrl Pts',(2.07642359732163,2.46470088149511,36.7343868019875));
#34596=CARTESIAN_POINT('Ctrl Pts',(2.0664993079806,2.47302769761647,36.735176696898));
#34597=CARTESIAN_POINT('Ctrl Pts',(2.04878125856672,2.48771262000182,36.7365842272608));
#34598=CARTESIAN_POINT('Ctrl Pts',(2.04100738834421,2.49409453755293,36.7372008800983));
#34599=CARTESIAN_POINT('Ctrl Pts',(2.02473884915917,2.50732311237492,36.7384895474435));
#34600=CARTESIAN_POINT('Ctrl Pts',(2.016239043971,2.51416322262954,36.7391618156184));
#34601=CARTESIAN_POINT('Ctrl Pts',(1.99405204187911,2.53183305872703,36.7409140909781));
#34602=CARTESIAN_POINT('Ctrl Pts',(1.9803114508983,2.54259487947004,36.7419967975236));
#34603=CARTESIAN_POINT('Ctrl Pts',(1.91997054415686,2.58906886700687,36.7467412015817));
#34604=CARTESIAN_POINT('Ctrl Pts',(1.87248916450982,2.62361355511462,36.7504484297529));
#34605=CARTESIAN_POINT('Ctrl Pts',(1.74328790330577,2.71231859679064,36.7604747270384));
#34606=CARTESIAN_POINT('Ctrl Pts',(1.66000072818877,2.76407660133745,36.7668766405699));
#34607=CARTESIAN_POINT('Ctrl Pts',(1.40766936111291,2.90536384818186,36.786061721988));
#34608=CARTESIAN_POINT('Ctrl Pts',(1.232871877232,2.9837377322838,36.7991106145913));
#34609=CARTESIAN_POINT('Ctrl Pts',(0.926532175384797,3.08955104591862,36.8209196403535));
#34610=CARTESIAN_POINT('Ctrl Pts',(0.798307190894622,3.12514024818465,36.8297459469964));
#34611=CARTESIAN_POINT('Ctrl Pts',(0.653620244386708,3.15580756373062,36.8391233165872));
#34612=CARTESIAN_POINT('Ctrl Pts',(0.638982021735399,3.15880401407526,36.8400654689786));
#34613=CARTESIAN_POINT('Ctrl Pts',(0.617276612328088,3.16309006136898,36.8414522305245));
#34614=CARTESIAN_POINT('Ctrl Pts',(0.610225350643649,3.16445795931336,36.8419011387716));
#34615=CARTESIAN_POINT('Ctrl Pts',(0.597677836891366,3.1668485942409,36.8426970460851));
#34616=CARTESIAN_POINT('Ctrl Pts',(0.592183448714921,3.16788061333103,36.8430445684284));
#34617=CARTESIAN_POINT('Ctrl Pts',(0.58036448649849,3.17006876268273,36.8437899708233));
#34618=CARTESIAN_POINT('Ctrl Pts',(0.574039147667095,3.17122026292387,36.8441875851245));
#34619=CARTESIAN_POINT('Ctrl Pts',(0.55656201494484,3.17434789388611,36.8452826853262));
#34620=CARTESIAN_POINT('Ctrl Pts',(0.545403057365658,3.17628420356421,36.8459779394641));
#34621=CARTESIAN_POINT('Ctrl Pts',(0.48400431868569,3.18660504084151,36.8497827884402));
#34622=CARTESIAN_POINT('Ctrl Pts',(0.433578292551593,3.19385697964606,36.8528320604096));
#34623=CARTESIAN_POINT('Ctrl Pts',(0.126694374032891,3.23058801392747,36.8710472475619));
#34624=CARTESIAN_POINT('Ctrl Pts',(-0.132392916066827,3.23036419740347,
36.8850459308302));
#34625=CARTESIAN_POINT('Ctrl Pts',(-0.553144886143904,3.17924354978906,
36.9089761751536));
#34626=CARTESIAN_POINT('Ctrl Pts',(-0.715783007048575,3.14661767538846,
36.9185165948688));
#34627=CARTESIAN_POINT('Ctrl Pts',(-0.896295515390018,3.09568300091237,
36.9297975036102));
#34628=CARTESIAN_POINT('Ctrl Pts',(-0.917348495585595,3.08950976600439,
36.931123803746));
#34629=CARTESIAN_POINT('Ctrl Pts',(-0.950871975286829,3.07930702346509,
36.9332534381652));
#34630=CARTESIAN_POINT('Ctrl Pts',(-0.963384003351651,3.07541550237927,
36.9340522528097));
#34631=CARTESIAN_POINT('Ctrl Pts',(-0.985479219561552,3.06839532825165,
36.9354700707615));
#34632=CARTESIAN_POINT('Ctrl Pts',(-0.995072167840309,3.06529779299603,
36.9360880416007));
#34633=CARTESIAN_POINT('Ctrl Pts',(-1.01495353803362,3.05877499347314,36.9373738543905));
#34634=CARTESIAN_POINT('Ctrl Pts',(-1.02523950770585,3.05534271274126,36.9380419221032));
#34635=CARTESIAN_POINT('Ctrl Pts',(-1.05174915691184,3.04634788252861,36.9397711234567));
#34636=CARTESIAN_POINT('Ctrl Pts',(-1.06794594537064,3.04070767254742,36.940834825075));
#34637=CARTESIAN_POINT('Ctrl Pts',(-1.13673876207206,3.01613450103769,36.9453839773432));
#34638=CARTESIAN_POINT('Ctrl Pts',(-1.18887980529481,2.99596503961827,36.9489104514787));
#34639=CARTESIAN_POINT('Ctrl Pts',(-1.32490043599684,2.93923888201575,36.958324879121));
#34640=CARTESIAN_POINT('Ctrl Pts',(-1.40778887040859,2.90045072006253,36.9642836859241));
#34641=CARTESIAN_POINT('Ctrl Pts',(-1.70772472929498,2.74420604356364,36.9866514534945));
#34642=CARTESIAN_POINT('Ctrl Pts',(-1.91270368009395,2.60548260354482,37.0036323679565));
#34643=CARTESIAN_POINT('Ctrl Pts',(-2.16733902784523,2.38677102064044,37.0259392947688));
#34644=CARTESIAN_POINT('Ctrl Pts',(-2.23241276480209,2.32602036633145,37.0317570263363));
#34645=CARTESIAN_POINT('Ctrl Pts',(-2.30459826389271,2.25280612658301,37.0382686764267));
#34646=CARTESIAN_POINT('Ctrl Pts',(-2.3142390779141,2.24290127029268,37.0391395910877));
#34647=CARTESIAN_POINT('Ctrl Pts',(-2.32870215248365,2.22784954115069,37.0404475897907));
#34648=CARTESIAN_POINT('Ctrl Pts',(-2.33357158612701,2.22274851201286,37.0408882204375));
#34649=CARTESIAN_POINT('Ctrl Pts',(-2.34226356460735,2.2135830876514,37.0416751359755));
#34650=CARTESIAN_POINT('Ctrl Pts',(-2.346092319323,2.20952472780483,37.0420218979329));
#34651=CARTESIAN_POINT('Ctrl Pts',(-2.35437302294139,2.2007016498423,37.0427721404088));
#34652=CARTESIAN_POINT('Ctrl Pts',(-2.3588210427999,2.19593337162044,37.0431753205467));
#34653=CARTESIAN_POINT('Ctrl Pts',(-2.37123931686889,2.18253970971524,37.0443015737209));
#34654=CARTESIAN_POINT('Ctrl Pts',(-2.37917703781714,2.17388410798806,37.0450222011656));
#34655=CARTESIAN_POINT('Ctrl Pts',(-2.42573118851716,2.12255921522773,37.0492543391556));
#34656=CARTESIAN_POINT('Ctrl Pts',(-2.46324908445984,2.07890219088969,37.0526884271842));
#34657=CARTESIAN_POINT('Ctrl Pts',(-2.65930140451222,1.83800460723727,37.0709110177983));
#34658=CARTESIAN_POINT('Ctrl Pts',(-2.79536817759413,1.62360345248578,37.0846448609797));
#34659=CARTESIAN_POINT('Ctrl Pts',(-2.97573333399933,1.24813681637361,37.1081755874179));
#34660=CARTESIAN_POINT('Ctrl Pts',(-3.03518938676924,1.09565021399464,37.1175957507025));
#34661=CARTESIAN_POINT('Ctrl Pts',(-3.08920302742152,0.918379895379297,
37.1287420858921));
#34662=CARTESIAN_POINT('Ctrl Pts',(-3.09537110838261,0.897370961205556,
37.1300657795763));
#34663=CARTESIAN_POINT('Ctrl Pts',(-3.10488397570805,0.863703896920118,
37.1321920182396));
#34664=CARTESIAN_POINT('Ctrl Pts',(-3.10836660299303,0.851085176480857,
37.1329900665771));
#34665=CARTESIAN_POINT('Ctrl Pts',(-3.11439433102335,0.828714120288518,
37.1344069975532));
#34666=CARTESIAN_POINT('Ctrl Pts',(-3.11697075770407,0.818970350030057,
37.1350248520166));
#34667=CARTESIAN_POINT('Ctrl Pts',(-3.12222555820101,0.798713233184525,
37.1363108945144));
#34668=CARTESIAN_POINT('Ctrl Pts',(-3.12489663064067,0.788198140285589,
37.1369793106554));
#34669=CARTESIAN_POINT('Ctrl Pts',(-3.13165917973631,0.761001547505315,
37.1387104280406));
#34670=CARTESIAN_POINT('Ctrl Pts',(-3.13567044260096,0.744300631681173,
37.1397757080816));
#34671=CARTESIAN_POINT('Ctrl Pts',(-3.15221945776199,0.672889607208716,
37.1443407616012));
#34672=CARTESIAN_POINT('Ctrl Pts',(-3.16345965886952,0.617891803538932,
37.1478819161826));
#34673=CARTESIAN_POINT('Ctrl Pts',(-3.18931977790645,0.472039927098291,
37.1573454942228));
#34674=CARTESIAN_POINT('Ctrl Pts',(-3.20149397223313,0.380809869881011,
37.1633396944617));
#34675=CARTESIAN_POINT('Ctrl Pts',(-3.23146072734248,0.0482064408569172,
37.1854324681332));
#34676=CARTESIAN_POINT('Ctrl Pts',(-3.22596406277041,-0.194430714669504,
37.2020723137423));
#34677=CARTESIAN_POINT('Ctrl Pts',(-3.18088225099349,-0.526024420256396,
37.22434190437));
#34678=CARTESIAN_POINT('Ctrl Pts',(-3.16443211676231,-0.617321996036819,
37.2304125155196));
#34679=CARTESIAN_POINT('Ctrl Pts',(-3.14100181686343,-0.721401250402509,
37.2371701970664));
#34680=CARTESIAN_POINT('Ctrl Pts',(-3.13784956707135,-0.734991352746937,
37.238049324232));
#34681=CARTESIAN_POINT('Ctrl Pts',(-3.13296472537972,-0.755446696316358,
37.2393671989953));
#34682=CARTESIAN_POINT('Ctrl Pts',(-3.1312976444493,-0.762327190639459,
37.2398095715792));
#34683=CARTESIAN_POINT('Ctrl Pts',(-3.12827571303548,-0.774622345565591,
37.24059836306));
#34684=CARTESIAN_POINT('Ctrl Pts',(-3.12692946109608,-0.780039013078377,
37.240945268769));
#34685=CARTESIAN_POINT('Ctrl Pts',(-3.12398479059021,-0.791756810987841,
37.2416944183312));
#34686=CARTESIAN_POINT('Ctrl Pts',(-3.1223813824102,-0.798056592057209,
37.242096369373));
#34687=CARTESIAN_POINT('Ctrl Pts',(-3.11785094746984,-0.815633975101017,
37.243215721764));
#34688=CARTESIAN_POINT('Ctrl Pts',(-3.11488177370662,-0.826900754306286,
37.2439307256483));
#34689=CARTESIAN_POINT('Ctrl Pts',(-3.09728790003992,-0.89222251294425,
37.2480630269886));
#34690=CARTESIAN_POINT('Ctrl Pts',(-3.08131642639808,-0.945908721459504,
37.2514070996175));
#34691=CARTESIAN_POINT('Ctrl Pts',(-2.98515110660766,-1.24080389563577,
37.2696241341481));
#34692=CARTESIAN_POINT('Ctrl Pts',(-2.87803202414719,-1.47230447864389,
37.2834171147081));
#34693=CARTESIAN_POINT('Ctrl Pts',(-2.65885976161363,-1.82851934396009,
37.3070405146908));
#34694=CARTESIAN_POINT('Ctrl Pts',(-2.56238400196479,-1.96142702769182,
37.3164913659328));
#34695=CARTESIAN_POINT('Ctrl Pts',(-2.44203953090745,-2.10310256496634,
37.3276720280684));
#34696=CARTESIAN_POINT('Ctrl Pts',(-2.42768750438157,-2.11965346555868,
37.328996392058));
#34697=CARTESIAN_POINT('Ctrl Pts',(-2.40448948106646,-2.14586097999958,
37.3311235040547));
#34698=CARTESIAN_POINT('Ctrl Pts',(-2.39575127014583,-2.15561240804024,
37.3319217495112));
#34699=CARTESIAN_POINT('Ctrl Pts',(-2.3801819403947,-2.17277543323153,37.3333389085882));
#34700=CARTESIAN_POINT('Ctrl Pts',(-2.37337498200137,-2.18020878444696,
37.3339567929294));
#34701=CARTESIAN_POINT('Ctrl Pts',(-2.35916991163932,-2.19557567899414,
37.3352427760587));
#34702=CARTESIAN_POINT('Ctrl Pts',(-2.35176639903119,-2.20350403538454,
37.3359111023494));
#34703=CARTESIAN_POINT('Ctrl Pts',(-2.33254173034325,-2.2238843106004,37.3376417256947));
#34704=CARTESIAN_POINT('Ctrl Pts',(-2.3206609577078,-2.23627928750168,37.3387065987548));
#34705=CARTESIAN_POINT('Ctrl Pts',(-2.26956127909485,-2.28874483413571,
37.3432675469909));
#34706=CARTESIAN_POINT('Ctrl Pts',(-2.22940126084228,-2.32788116026025,
37.3468049107828));
#34707=CARTESIAN_POINT('Ctrl Pts',(-2.12079814275964,-2.4283271441839,37.3562557881338));
#34708=CARTESIAN_POINT('Ctrl Pts',(-2.05072260321249,-2.48778852983414,
37.3622408391819));
#34709=CARTESIAN_POINT('Ctrl Pts',(-1.82076289780361,-2.66659256755328,
37.3815103996241));
#34710=CARTESIAN_POINT('Ctrl Pts',(-1.65238201600226,-2.77406600268191,
37.3951166831969));
#34711=CARTESIAN_POINT('Ctrl Pts',(-1.47525540431025,-2.86526422072266,
37.4085260041042));
#34712=CARTESIAN_POINT('Origin',(0.,0.,4.68922655072688));
#34713=CARTESIAN_POINT('',(-1.47525540501186,-2.86526422036142,34.9999952908233));
#34714=CARTESIAN_POINT('',(-1.47525552646581,-2.8652641578277,35.1563175586878));
#34715=CARTESIAN_POINT('',(-1.47525540501186,-2.86526422036142,4.68922655072688));
#34716=CARTESIAN_POINT('',(-3.05037901532684,-1.03985836792983,35.0000143649096));
#34717=CARTESIAN_POINT('Origin',(0.,0.,35.));
#34718=CARTESIAN_POINT('Ctrl Pts',(-1.47525552646581,-2.8652641578277,35.1563175586878));
#34719=CARTESIAN_POINT('Ctrl Pts',(-1.5179786368742,-2.84326705694414,35.1534900287168));
#34720=CARTESIAN_POINT('Ctrl Pts',(-1.56021632410078,-2.82031103518203,
35.150632229143));
#34721=CARTESIAN_POINT('Ctrl Pts',(-1.62096631363004,-2.78551014190289,
35.146421317202));
#34722=CARTESIAN_POINT('Ctrl Pts',(-1.63988409403924,-2.7744150126229,35.1450954968172));
#34723=CARTESIAN_POINT('Ctrl Pts',(-1.6699213053194,-2.75638387962761,35.1429663459599));
#34724=CARTESIAN_POINT('Ctrl Pts',(-1.68111443427663,-2.74957151366147,
35.1421675300128));
#34725=CARTESIAN_POINT('Ctrl Pts',(-1.70084704537755,-2.73739631176315,
35.1407495369148));
#34726=CARTESIAN_POINT('Ctrl Pts',(-1.70940353540863,-2.73206127107097,
35.1401313914053));
#34727=CARTESIAN_POINT('Ctrl Pts',(-1.72711415399747,-2.72090278595853,
35.1388450421301));
#34728=CARTESIAN_POINT('Ctrl Pts',(-1.73626418293619,-2.71507310288679,
35.1381766115914));
#34729=CARTESIAN_POINT('Ctrl Pts',(-1.75981505434774,-2.69990059222446,
35.1364460971715));
#34730=CARTESIAN_POINT('Ctrl Pts',(-1.77417085675511,-2.6904888005836,35.135381439547));
#34731=CARTESIAN_POINT('Ctrl Pts',(-1.83503964978362,-2.64988367822589,
35.130824774063));
#34732=CARTESIAN_POINT('Ctrl Pts',(-1.88080814757814,-2.61759700897596,
35.1272915814473));
#34733=CARTESIAN_POINT('Ctrl Pts',(-1.99924781255354,-2.52933522155223,
35.1178552546094));
#34734=CARTESIAN_POINT('Ctrl Pts',(-2.07040678604797,-2.47142503715811,
35.1118808696354));
#34735=CARTESIAN_POINT('Ctrl Pts',(-2.32202096135386,-2.24815717635066,
35.0896297664439));
#34736=CARTESIAN_POINT('Ctrl Pts',(-2.48593682768389,-2.06545269928067,
35.0727943646564));
#34737=CARTESIAN_POINT('Ctrl Pts',(-2.68002016186566,-1.7921516345158,35.0505052130097));
#34738=CARTESIAN_POINT('Ctrl Pts',(-2.72931560658516,-1.71614543216571,
35.0445815800732));
#34739=CARTESIAN_POINT('Ctrl Pts',(-2.78240414784869,-1.62620336552493,
35.0379665134103));
#34740=CARTESIAN_POINT('Ctrl Pts',(-2.7893825488052,-1.61420421283992,35.037091854403));
#34741=CARTESIAN_POINT('Ctrl Pts',(-2.79979613030385,-1.59602917237582,
35.0357792620165));
#34742=CARTESIAN_POINT('Ctrl Pts',(-2.80328877516139,-1.58988664239112,
35.0353377469127));
#34743=CARTESIAN_POINT('Ctrl Pts',(-2.80950444728965,-1.57887095232093,
35.0345497698746));
#34744=CARTESIAN_POINT('Ctrl Pts',(-2.81223503144743,-1.574002176899,35.0342028264667));
#34745=CARTESIAN_POINT('Ctrl Pts',(-2.81812494196711,-1.5634359004169,35.0334527747247));
#34746=CARTESIAN_POINT('Ctrl Pts',(-2.82127963779431,-1.55773592447216,
35.0330499638339));
#34747=CARTESIAN_POINT('Ctrl Pts',(-2.83005619289586,-1.54176412620451,
35.0319261826464));
#34748=CARTESIAN_POINT('Ctrl Pts',(-2.83563945374104,-1.53147104902214,
35.0312076395943));
#34749=CARTESIAN_POINT('Ctrl Pts',(-2.86803336675817,-1.47096639833774,
35.0270157530493));
#34750=CARTESIAN_POINT('Ctrl Pts',(-2.89356790136217,-1.42007861040143,
35.0236181149031));
#34751=CARTESIAN_POINT('Ctrl Pts',(-2.96799167462051,-1.26140600856599,
35.0133313483208));
#34752=CARTESIAN_POINT('Ctrl Pts',(-3.01226077392425,-1.15167656092768,
35.0066413036545));
#34753=CARTESIAN_POINT('Ctrl Pts',(-3.05037901532683,-1.03985836792984,
35.0000143649095));
#34754=CARTESIAN_POINT('Ctrl Pts',(1.43039598794072,-2.88162839993989,6.58668234580631));
#34755=CARTESIAN_POINT('Ctrl Pts',(2.3908869304735,-2.40485547853165,6.65299332526079));
#34756=CARTESIAN_POINT('Ctrl Pts',(3.78068485083689,-0.42330470969778,6.78561528416975));
#34757=CARTESIAN_POINT('Ctrl Pts',(2.39660828659712,2.9593008547868,6.98454822253319));
#34758=CARTESIAN_POINT('Ctrl Pts',(-1.19393826692811,3.61225397709376,7.18348116089663));
#34759=CARTESIAN_POINT('Ctrl Pts',(-3.68522155716544,0.949002744436199,
7.38241409926007));
#34760=CARTESIAN_POINT('Ctrl Pts',(-2.78953196244949,-2.58902355773568,
7.5813470376235));
#34761=CARTESIAN_POINT('Ctrl Pts',(0.671039291373588,-3.74572463321816,
7.78027997598695));
#34762=CARTESIAN_POINT('Ctrl Pts',(3.51448527473695,-1.45960212386322,7.97921291435037));
#34763=CARTESIAN_POINT('Ctrl Pts',(3.12717197768531,2.16867191230057,8.17814585271383));
#34764=CARTESIAN_POINT('Ctrl Pts',(-0.135028807280012,3.80310255787661,
8.37707879107726));
#34765=CARTESIAN_POINT('Ctrl Pts',(-3.27306356366253,1.94141424541036,8.5760117294407));
#34766=CARTESIAN_POINT('Ctrl Pts',(-3.40217358758694,-1.70507215059562,
8.77494466780414));
#34767=CARTESIAN_POINT('Ctrl Pts',(-0.403640923403273,-3.78405339475958,
8.97387760616759));
#34768=CARTESIAN_POINT('Ctrl Pts',(2.96595593022244,-2.38435003081143,9.172810544531));
#34769=CARTESIAN_POINT('Ctrl Pts',(3.60893852822567,1.20730380998424,9.37174348289446));
#34770=CARTESIAN_POINT('Ctrl Pts',(0.934206293343398,3.68907429945195,9.57067642125789));
#34771=CARTESIAN_POINT('Ctrl Pts',(-2.59934534842778,2.77946388606067,9.76960935962134));
#34772=CARTESIAN_POINT('Ctrl Pts',(-3.7433073822935,-0.685321221973841,
9.96854229798476));
#34773=CARTESIAN_POINT('Ctrl Pts',(-1.4460297930754,-3.52008693042821,10.1674752363482));
#34774=CARTESIAN_POINT('Ctrl Pts',(2.18058944266648,-3.11882102941849,10.3664081747117));
#34775=CARTESIAN_POINT('Ctrl Pts',(3.80258297155867,0.14959131214445,10.5653411130751));
#34776=CARTESIAN_POINT('Ctrl Pts',(1.92884471639216,3.28048361242447,10.7642740514386));
#34777=CARTESIAN_POINT('Ctrl Pts',(-1.71808921409888,3.39561249800469,10.963206989802));
#34778=CARTESIAN_POINT('Ctrl Pts',(-3.78557595114969,0.389139407006486,
11.1621399281654));
#34779=CARTESIAN_POINT('Ctrl Pts',(-2.37296555731667,-2.97507129439684,
11.3610728665289));
#34780=CARTESIAN_POINT('Ctrl Pts',(1.2211228251491,-3.60428547773973,11.5600058048923));
#34781=CARTESIAN_POINT('Ctrl Pts',(3.69262746162031,-0.920063684940536,
11.7589387432558));
#34782=CARTESIAN_POINT('Ctrl Pts',(2.76948293800576,2.60997682152157,11.9578716816192));
#34783=CARTESIAN_POINT('Ctrl Pts',(-0.699659800874596,3.74065380890841,
12.1568046199826));
#34784=CARTESIAN_POINT('Ctrl Pts',(-3.52560211426312,1.43253079764144,12.3557375583461));
#34785=CARTESIAN_POINT('Ctrl Pts',(-3.11044242675709,-2.19252426758155,
12.5546704967095));
#34786=CARTESIAN_POINT('Ctrl Pts',(0.164161079403195,-3.8019818377298,12.7536034350729));
#34787=CARTESIAN_POINT('Ctrl Pts',(3.2878505613498,-1.91626027473385,12.9525363734364));
#34788=CARTESIAN_POINT('Ctrl Pts',(3.38900412249117,1.73108804282604,13.1514693117998));
#34789=CARTESIAN_POINT('Ctrl Pts',(0.374630835682455,3.78703927775718,13.3504022501632));
#34790=CARTESIAN_POINT('Ctrl Pts',(-2.98414227610861,2.36154814268967,13.5493351885267));
#34791=CARTESIAN_POINT('Ctrl Pts',(-3.59957987005836,-1.23492490191512,
13.7482681268901));
#34792=CARTESIAN_POINT('Ctrl Pts',(-0.905907377036315,-3.69612588780959,
13.9472010652536));
#34793=CARTESIAN_POINT('Ctrl Pts',(2.6205698730494,-2.7594615950884,14.146134003617));
#34794=CARTESIAN_POINT('Ctrl Pts',(3.73794536304987,0.713988247211487,14.3450669419804));
#34795=CARTESIAN_POINT('Ctrl Pts',(1.41901074133174,3.53106545822759,14.5439998803439));
#34796=CARTESIAN_POINT('Ctrl Pts',(-2.2044268855072,3.10201819155779,14.7429328187073));
#34797=CARTESIAN_POINT('Ctrl Pts',(-3.8013248865683,-0.178728456209389,
14.9418657570708));
#34798=CARTESIAN_POINT('Ctrl Pts',(-1.90364769271949,-3.29516922422906,
15.1407986954342));
#34799=CARTESIAN_POINT('Ctrl Pts',(1.74406145191863,-3.38234599150264,15.3397316337976));
#34800=CARTESIAN_POINT('Ctrl Pts',(3.78844700014203,-0.360116760811474,
15.5386645721611));
#34801=CARTESIAN_POINT('Ctrl Pts',(2.35009605280664,2.993169440056,15.7375975105245));
#34802=CARTESIAN_POINT('Ctrl Pts',(-1.24870884594248,3.59482141035789,15.9365304488879));
#34803=CARTESIAN_POINT('Ctrl Pts',(-3.69957004376932,0.891737767254035,
16.1354633872514));
#34804=CARTESIAN_POINT('Ctrl Pts',(-2.74939973479973,-2.63112444642698,
16.3343963256148));
#34805=CARTESIAN_POINT('Ctrl Pts',(0.728306209987826,-3.73518203288617,
16.5333292639783));
#34806=CARTESIAN_POINT('Ctrl Pts',(3.53647695542546,-1.40546984956888,16.7322622023417));
#34807=CARTESIAN_POINT('Ctrl Pts',(3.09354840927974,2.21629713570752,16.9311951407051));
#34808=CARTESIAN_POINT('Ctrl Pts',(-0.193293208732243,3.80061212040383,
17.1301280790686));
#34809=CARTESIAN_POINT('Ctrl Pts',(-3.30243950399845,1.89100715935529,17.329061017432));
#34810=CARTESIAN_POINT('Ctrl Pts',(-3.37563819737945,-1.75700925287699,
17.5279939557954));
#34811=CARTESIAN_POINT('Ctrl Pts',(-0.345597398331251,-3.78979909659722,
17.7269268941589));
#34812=CARTESIAN_POINT('Ctrl Pts',(3.00215265516693,-2.33860945636005,17.9258598325223));
#34813=CARTESIAN_POINT('Ctrl Pts',(3.5900101677383,1.26247445512302,18.1247927708858));
#34814=CARTESIAN_POINT('Ctrl Pts',(0.877555064047497,3.70295987878172,18.3237257092492));
#34815=CARTESIAN_POINT('Ctrl Pts',(-2.6416403868901,2.73929750495517,18.5226586476126));
#34816=CARTESIAN_POINT('Ctrl Pts',(-3.73236385888241,-0.742613479012362,
18.7215915859761));
#34817=CARTESIAN_POINT('Ctrl Pts',(-1.39190832123119,-3.54183652637864,
18.9205245243395));
#34818=CARTESIAN_POINT('Ctrl Pts',(2.22813484392072,-3.085033204296,19.119457462703));
#34819=CARTESIAN_POINT('Ctrl Pts',(3.79984354968653,0.20785512312247,19.3183904010664));
#34820=CARTESIAN_POINT('Ctrl Pts',(1.87833886025086,3.30966129390517,19.5173233394298));
#34821=CARTESIAN_POINT('Ctrl Pts',(-1.76993125559216,3.36888083861398,19.7162562777933));
#34822=CARTESIAN_POINT('Ctrl Pts',(-3.79109554726769,0.331072961429409,
19.9151892161567));
#34823=CARTESIAN_POINT('Ctrl Pts',(-2.32708852200922,-3.01109178954004,
20.1141221545202));
#34824=CARTESIAN_POINT('Ctrl Pts',(1.27622152733633,-3.58514621284347,20.3130550928836));
#34825=CARTESIAN_POINT('Ctrl Pts',(3.70629534307339,-0.863359475661814,
20.511988031247));
#34826=CARTESIAN_POINT('Ctrl Pts',(2.72915505388636,2.65211754003269,20.7109209696104));
#34827=CARTESIAN_POINT('Ctrl Pts',(-0.756909844210963,3.729490882418,20.9098539079739));
#34828=CARTESIAN_POINT('Ctrl Pts',(-3.54714409239226,1.37832635544315,21.1087868463373));
#34829=CARTESIAN_POINT('Ctrl Pts',(-3.07647270163572,-2.23993983633326,
21.3077197847008));
#34830=CARTESIAN_POINT('Ctrl Pts',(0.222413985566929,-3.79901918570132,
21.5066527230642));
#34831=CARTESIAN_POINT('Ctrl Pts',(3.31683448791136,-1.86564298141534,21.7055856614276));
#34832=CARTESIAN_POINT('Ctrl Pts',(3.36207401442483,1.78282727032986,21.9045185997911));
#34833=CARTESIAN_POINT('Ctrl Pts',(0.316543663368888,3.79233633311756,22.1034515381545));
#34834=CARTESIAN_POINT('Ctrl Pts',(-3.01998671192163,2.31553341891654,22.3023844765179));
#34835=CARTESIAN_POINT('Ctrl Pts',(-3.58022961709107,-1.28994986073349,
22.5013174148814));
#34836=CARTESIAN_POINT('Ctrl Pts',(-0.849151210531485,-3.70957638766954,
22.7002503532448));
#34837=CARTESIAN_POINT('Ctrl Pts',(2.66255575201821,-2.71897253051539,22.8991832916083));
#34838=CARTESIAN_POINT('Ctrl Pts',(3.72656314567699,0.771195095669392,23.0981162299717));
#34839=CARTESIAN_POINT('Ctrl Pts',(1.3647241516294,3.55239957553509,23.2970491683351));
#34840=CARTESIAN_POINT('Ctrl Pts',(-2.25171193961186,3.06786702699317,23.4959821066986));
#34841=CARTESIAN_POINT('Ctrl Pts',(-3.79813904055242,-0.236969582297126,
23.694915045062));
#34842=CARTESIAN_POINT('Ctrl Pts',(-1.85291970926293,-3.32395898069267,
23.8938479834255));
#34843=CARTESIAN_POINT('Ctrl Pts',(1.79569710773726,-3.35521782475692,24.0927809217889));
#34844=CARTESIAN_POINT('Ctrl Pts',(3.79352143592832,-0.302009717484061,
24.2917138601523));
#34845=CARTESIAN_POINT('Ctrl Pts',(2.30394431674614,3.02883729170711,24.4906467985158));
#34846=CARTESIAN_POINT('Ctrl Pts',(-1.30365925374081,3.57526045267173,24.6895797368792));
#34847=CARTESIAN_POINT('Ctrl Pts',(-3.71280296439449,0.834930477277034,
24.8885126752426));
#34848=CARTESIAN_POINT('Ctrl Pts',(-2.70875008435262,-2.67295486958203,
25.0874456136061));
#34849=CARTESIAN_POINT('Ctrl Pts',(0.785469023636781,-3.72358069164743,
25.2863785519695));
#34850=CARTESIAN_POINT('Ctrl Pts',(3.55760289864069,-1.35110190951161,25.485311490333));
#34851=CARTESIAN_POINT('Ctrl Pts',(3.05921630672578,2.26345098090627,25.6842444286964));
#34852=CARTESIAN_POINT('Ctrl Pts',(-0.251521699592702,3.79720312716301,
25.8831773670599));
#34853=CARTESIAN_POINT('Ctrl Pts',(-3.33103466763993,1.84016923060991,26.0821103054233));
#34854=CARTESIAN_POINT('Ctrl Pts',(-3.34831237027993,-1.80854057884607,
26.2810432437867));
#34855=CARTESIAN_POINT('Ctrl Pts',(-0.287471337177379,-3.79465083829908,
26.4799761821502));
#34856=CARTESIAN_POINT('Ctrl Pts',(3.03764339894311,-2.29232138566123,26.6789091205136));
#34857=CARTESIAN_POINT('Ctrl Pts',(3.57023879254785,1.31734950506271,26.877842058877));
#34858=CARTESIAN_POINT('Ctrl Pts',(0.820697484702102,3.71597502587224,27.0767749972405));
#34859=CARTESIAN_POINT('Ctrl Pts',(-2.68331474003338,2.69848786549469,27.2757079356039));
#34860=CARTESIAN_POINT('Ctrl Pts',(-3.72054356412085,-0.799731418528385,
27.4746408739674));
#34861=CARTESIAN_POINT('Ctrl Pts',(-1.3374598291058,-3.56275398530838,27.6735738123308));
#34862=CARTESIAN_POINT('Ctrl Pts',(2.27515678785163,-3.05052066785249,27.8725067506942));
#34863=CARTESIAN_POINT('Ctrl Pts',(3.79621145927515,0.266070123784241,28.0714396890576));
#34864=CARTESIAN_POINT('Ctrl Pts',(1.82739173267215,3.33806144486047,28.2703726274211));
#34865=CARTESIAN_POINT('Ctrl Pts',(-1.82135749507502,3.34135775238698,28.4693055657845));
#34866=CARTESIAN_POINT('Ctrl Pts',(-3.79572452364676,0.272928735916584,
28.668238504148));
#34867=CARTESIAN_POINT('Ctrl Pts',(-2.28066479632187,-3.04640490432913,
28.8671714425114));
#34868=CARTESIAN_POINT('Ctrl Pts',(1.33102041368457,-3.56516471045272,29.0661043808749));
#34869=CARTESIAN_POINT('Ctrl Pts',(3.71909252552727,-0.806452441790404,
29.2650373192383));
#34870=CARTESIAN_POINT('Ctrl Pts',(2.68818602462228,2.69363521125782,29.4639702576017));
#34871=CARTESIAN_POINT('Ctrl Pts',(-0.81398207092878,3.71745180769153,29.6629031959652));
#34872=CARTESIAN_POINT('Ctrl Pts',(-3.56785275990456,1.32379811071928,29.8618361343286));
#34873=CARTESIAN_POINT('Ctrl Pts',(-3.04178023805176,-2.286829188571,30.060769072692));
#34874=CARTESIAN_POINT('Ctrl Pts',(0.280614641256556,-3.79516405144956,
30.2597020110555));
#34875=CARTESIAN_POINT('Ctrl Pts',(3.34503920917982,-1.81458740306222,30.4586349494189));
#34876=CARTESIAN_POINT('Ctrl Pts',(3.33435407319303,1.83414766823269,30.6575678877823));
#34877=CARTESIAN_POINT('Ctrl Pts',(0.258382127231354,3.7967424762064,30.8565008261458));
#34878=CARTESIAN_POINT('Ctrl Pts',(-3.05512167921966,2.26897471988225,31.0554337645092));
#34879=CARTESIAN_POINT('Ctrl Pts',(-3.56003828088928,-1.34467177887595,
31.2543667028727));
#34880=CARTESIAN_POINT('Ctrl Pts',(-0.792195557702424,-3.7221554175852,
31.4532996412361));
#34881=CARTESIAN_POINT('Ctrl Pts',(2.70391613171949,-2.67784471299768,31.6522325795996));
#34882=CARTESIAN_POINT('Ctrl Pts',(3.71430546775585,0.828220771595132,31.851165517963));
#34883=CARTESIAN_POINT('Ctrl Pts',(1.31011695494754,3.57289914756372,32.0500984563264));
#34884=CARTESIAN_POINT('Ctrl Pts',(-2.29846801167811,3.03299514565962,32.2490313946898));
#34885=CARTESIAN_POINT('Ctrl Pts',(-3.79406091906533,-0.295155038451869,
32.4479643330533));
#34886=CARTESIAN_POINT('Ctrl Pts',(-1.8017564297867,-3.35196785814317,32.6468972714167));
#34887=CARTESIAN_POINT('Ctrl Pts',(1.84691091052057,-3.32730143553342,32.8458302097802));
#34888=CARTESIAN_POINT('Ctrl Pts',(3.79770468103133,-0.243831724710034,
33.0447631481436));
#34889=CARTESIAN_POINT('Ctrl Pts',(2.25725132798827,3.06379359562579,33.2436960865071));
#34890=CARTESIAN_POINT('Ctrl Pts',(-1.35830340019312,3.55485957912918,33.4426290248705));
#34891=CARTESIAN_POINT('Ctrl Pts',(-3.72516365707354,0.777927041772669,
33.6415619632339));
#34892=CARTESIAN_POINT('Ctrl Pts',(-2.66746408246281,-2.71415735046314,
33.8404949015973));
#34893=CARTESIAN_POINT('Ctrl Pts',(0.842447311459858,-3.71110459051167,
34.0394278399608));
#34894=CARTESIAN_POINT('Ctrl Pts',(3.57789307418948,-1.29641656267163,34.2383607783242));
#34895=CARTESIAN_POINT('Ctrl Pts',(3.02416551966811,2.31007308627943,34.4372937166877));
#34896=CARTESIAN_POINT('Ctrl Pts',(-0.309691101873131,3.79290207832017,
34.6362266550511));
#34897=CARTESIAN_POINT('Ctrl Pts',(-3.35884729001673,1.78889900124255,34.8351595934145));
#34898=CARTESIAN_POINT('Ctrl Pts',(-3.32019994296254,-1.85964703453407,
35.034092531778));
#34899=CARTESIAN_POINT('Ctrl Pts',(-0.229277741996502,-3.79861112399583,
35.2330254701414));
#34900=CARTESIAN_POINT('Ctrl Pts',(3.07242052621671,-2.24549479277051,35.4319584085049));
#34901=CARTESIAN_POINT('Ctrl Pts',(3.54962868121306,1.37191507747408,35.6308913468683));
#34902=CARTESIAN_POINT('Ctrl Pts',(0.763647103503218,3.72811719983819,35.8298242852317));
#34903=CARTESIAN_POINT('Ctrl Pts',(-2.72435871711047,2.65704428540604,36.0287572235952));
#34904=CARTESIAN_POINT('Ctrl Pts',(-3.70784922296926,-0.856661481574834,
36.2276901619586));
#34905=CARTESIAN_POINT('Ctrl Pts',(-1.28269713503262,-3.58283446656971,
36.426623100322));
#34906=CARTESIAN_POINT('Ctrl Pts',(2.3216442419344,-3.01529148950444,36.6255560386855));
#34907=CARTESIAN_POINT('Ctrl Pts',(3.79168754631124,0.324222617667434,36.8244889770489));
#34908=CARTESIAN_POINT('Ctrl Pts',(1.77601530605909,3.36567740459321,37.0234219154124));
#34909=CARTESIAN_POINT('Ctrl Pts',(-1.8723558529673,3.31304969821073,37.2223548537758));
#34910=CARTESIAN_POINT('Ctrl Pts',(-3.7994617923675,0.214720395742962,37.4212877921392));
#34911=CARTESIAN_POINT('Ctrl Pts',(-2.23370528574428,-3.08100234999048,
37.6202207305027));
#34912=CARTESIAN_POINT('Ctrl Pts',(1.38550660873585,-3.54434565307739,37.8191536688661));
#34913=CARTESIAN_POINT('Ctrl Pts',(3.73101600658191,-0.749355973410843,
38.0180866072295));
#34914=CARTESIAN_POINT('Ctrl Pts',(2.64658546701708,2.7345201218469,38.217019545593));
#34915=CARTESIAN_POINT('Ctrl Pts',(-0.870863058265686,3.70453933627131,
38.4159524839564));
#34916=CARTESIAN_POINT('Ctrl Pts',(-3.58772328085212,1.26895902047793,38.6148854223199));
#34917=CARTESIAN_POINT('Ctrl Pts',(-3.00637313042353,-2.33318159065596,
38.8138183606833));
#34918=CARTESIAN_POINT('Ctrl Pts',(0.338749266911483,-3.79041680024323,
39.0127512990467));
#34919=CARTESIAN_POINT('Ctrl Pts',(3.37245830401273,-1.76310657017941,39.2116842374102));
#34920=CARTESIAN_POINT('Ctrl Pts',(3.30585041806794,1.88503916744779,39.4106171757737));
#34921=CARTESIAN_POINT('Ctrl Pts',(0.200160644147806,3.80025286079382,39.609550114137));
#34922=CARTESIAN_POINT('Ctrl Pts',(-3.08954036858721,2.2218902919993,39.8084830525005));
#34923=CARTESIAN_POINT('Ctrl Pts',(-3.53900783447175,-1.39909181671731,
40.0074159908639));
#34924=CARTESIAN_POINT('Ctrl Pts',(-0.735059111694563,-3.73383314394713,
40.2063489292274));
#34925=CARTESIAN_POINT('Ctrl Pts',(2.74465148416864,-2.63613934982058,40.4052818675907));
#34926=CARTESIAN_POINT('Ctrl Pts',(3.70115567014427,0.885150728230919,40.6042148059543));
#34927=CARTESIAN_POINT('Ctrl Pts',(1.25523944945949,3.59236978650378,40.8031477443176));
#34928=CARTESIAN_POINT('Ctrl Pts',(-2.34475597191911,2.99777433843635,41.0020806826812));
#34929=CARTESIAN_POINT('Ctrl Pts',(-3.78895369938313,-0.353968922753305,
41.2010136210445));
#34930=CARTESIAN_POINT('Ctrl Pts',(-1.75043395750614,-3.37784670177234,
41.399946559408));
#34931=CARTESIAN_POINT('Ctrl Pts',(1.89819598814578,-3.30121868695718,41.5988794977715));
#34932=CARTESIAN_POINT('Ctrl Pts',(3.80045064895368,-0.179534356723371,
41.7978556019462));
#34933=CARTESIAN_POINT('Ctrl Pts',(2.74058008982409,1.99769120286346,41.9305207266665));
#34934=CARTESIAN_POINT('Ctrl Pts',(1.86660756886202,2.62022723339283,41.9968748719324));
#34935=CARTESIAN_POINT('Ctrl Pts',(1.53698740838146,-3.09636394654476,6.72509367227838));
#34936=CARTESIAN_POINT('Ctrl Pts',(2.56905300209345,-2.58406246986299,6.79140465173286));
#34937=CARTESIAN_POINT('Ctrl Pts',(4.06241702282764,-0.454848876953752,
6.92402661064182));
#34938=CARTESIAN_POINT('Ctrl Pts',(2.5752007069213,3.17982446103466,7.12295954900526));
#34939=CARTESIAN_POINT('Ctrl Pts',(-1.28290913713704,3.88143487920559,7.32189248736869));
#34940=CARTESIAN_POINT('Ctrl Pts',(-3.9598399172061,1.01972130865502,7.52082542573213));
#34941=CARTESIAN_POINT('Ctrl Pts',(-2.9974045912523,-2.78195453691917,7.71975836409557));
#34942=CARTESIAN_POINT('Ctrl Pts',(0.721044347205764,-4.02485161106244,
7.91869130245901));
#34943=CARTESIAN_POINT('Ctrl Pts',(3.776380568565,-1.56836995107503,8.11762424082243));
#34944=CARTESIAN_POINT('Ctrl Pts',(3.36020514183989,2.33027878309083,8.3165571791859));
#34945=CARTESIAN_POINT('Ctrl Pts',(-0.145090994597224,4.08650527093188,
8.51549011754931));
#34946=CARTESIAN_POINT('Ctrl Pts',(-3.51696839657934,2.08608614314127,8.71442305591277));
#34947=CARTESIAN_POINT('Ctrl Pts',(-3.65569954707234,-1.83213211442255,
8.91335599427619));
#34948=CARTESIAN_POINT('Ctrl Pts',(-0.433719768517655,-4.06603658666688,
9.11228893263964));
#34949=CARTESIAN_POINT('Ctrl Pts',(3.18697546483547,-2.5620289803853,9.31122187100306));
#34950=CARTESIAN_POINT('Ctrl Pts',(3.87787236700172,1.2972706646837,9.51015480936652));
#34951=CARTESIAN_POINT('Ctrl Pts',(1.00382224349398,3.96397976129963,9.70908774772995));
#34952=CARTESIAN_POINT('Ctrl Pts',(-2.7930454952688,2.98658625369632,9.90802068609338));
#34953=CARTESIAN_POINT('Ctrl Pts',(-4.02225422945243,-0.736390550414543,
10.1069536244569));
#34954=CARTESIAN_POINT('Ctrl Pts',(-1.55378622621903,-3.78239965302563,
10.3058865628203));
#34955=CARTESIAN_POINT('Ctrl Pts',(2.34308439375097,-3.3512318907665,10.5048195011837));
#34956=CARTESIAN_POINT('Ctrl Pts',(4.08594696565489,0.160738680133138,10.7037524395472));
#34957=CARTESIAN_POINT('Ctrl Pts',(2.07257994765896,3.52494137861565,10.9026853779106));
#34958=CARTESIAN_POINT('Ctrl Pts',(-1.84611919413145,3.64864953283978,11.101618316274));
#34959=CARTESIAN_POINT('Ctrl Pts',(-4.06767260216181,0.418137616238003,
11.3005512546375));
#34960=CARTESIAN_POINT('Ctrl Pts',(-2.54979614936507,-3.19677009518745,
11.4994841930009));
#34961=CARTESIAN_POINT('Ctrl Pts',(1.31211945654531,-3.87287257668649,11.6984171313644));
#34962=CARTESIAN_POINT('Ctrl Pts',(3.96779770091828,-0.98862574460827,11.8973500697278));
#34963=CARTESIAN_POINT('Ctrl Pts',(2.97586153717486,2.80446921318709,12.0962830080912));
#34964=CARTESIAN_POINT('Ctrl Pts',(-0.75179762328831,4.01940291491122,12.2952159464547));
#34965=CARTESIAN_POINT('Ctrl Pts',(-3.78832582184925,1.53928130158088,12.4941488848181));
#34966=CARTESIAN_POINT('Ctrl Pts',(-3.34222892452571,-2.35590858772967,
12.6930818231815));
#34967=CARTESIAN_POINT('Ctrl Pts',(0.176394169248418,-4.08530103604272,
12.892014761545));
#34968=CARTESIAN_POINT('Ctrl Pts',(3.53285730387823,-2.05905772826418,13.0909476999084));
#34969=CARTESIAN_POINT('Ctrl Pts',(3.64154870898418,1.86008668023026,13.2898806382719));
#34970=CARTESIAN_POINT('Ctrl Pts',(0.402547883306248,4.06924497414062,13.4888135766353));
#34971=CARTESIAN_POINT('Ctrl Pts',(-3.20651703574811,2.53752792247832,13.6877465149988));
#34972=CARTESIAN_POINT('Ctrl Pts',(-3.86781631267568,-1.32695004777861,
13.8866794533622));
#34973=CARTESIAN_POINT('Ctrl Pts',(-0.973414525350525,-3.97155682569729,
14.0856123917256));
#34974=CARTESIAN_POINT('Ctrl Pts',(2.81585164640969,-2.96509341561348,14.284545330089));
#34975=CARTESIAN_POINT('Ctrl Pts',(4.01649263886463,0.767193808531516,14.4834782684525));
#34976=CARTESIAN_POINT('Ctrl Pts',(1.52475374663538,3.79419628775648,14.6824112068159));
#34977=CARTESIAN_POINT('Ctrl Pts',(-2.36869817469211,3.33317692526415,14.8813441451794));
#34978=CARTESIAN_POINT('Ctrl Pts',(-4.08459512965621,-0.192047089777438,
15.0802770835428));
#34979=CARTESIAN_POINT('Ctrl Pts',(-2.04550527152725,-3.54072134487557,
15.2792100219063));
#34980=CARTESIAN_POINT('Ctrl Pts',(1.87402685245334,-3.63439442193429,15.4781429602697));
#34981=CARTESIAN_POINT('Ctrl Pts',(4.07075759833579,-0.386952236709728,
15.6770758986331));
#34982=CARTESIAN_POINT('Ctrl Pts',(2.52522243637638,3.21621689329631,15.8760088369966));
#34983=CARTESIAN_POINT('Ctrl Pts',(-1.34176115504296,3.86270325817569,16.07494177536));
#34984=CARTESIAN_POINT('Ctrl Pts',(-3.97525763609332,0.958189012974472,
16.2738747137235));
#34985=CARTESIAN_POINT('Ctrl Pts',(-2.95428175737412,-2.8271927341357,16.4728076520868));
#34986=CARTESIAN_POINT('Ctrl Pts',(0.782578728991608,-4.01352338859924,
16.6717405904503));
#34987=CARTESIAN_POINT('Ctrl Pts',(3.80001104333727,-1.51020380360336,16.8706735288137));
#34988=CARTESIAN_POINT('Ctrl Pts',(3.3240759848093,2.38145298192455,17.0696064671772));
#34989=CARTESIAN_POINT('Ctrl Pts',(-0.207697190464619,4.08382924899859,
17.2685394055406));
#34990=CARTESIAN_POINT('Ctrl Pts',(-3.54853339731083,2.03192278053888,17.4674723439041));
#34991=CARTESIAN_POINT('Ctrl Pts',(-3.62718677091157,-1.88793950825425,
17.6664052822675));
#34992=CARTESIAN_POINT('Ctrl Pts',(-0.37135090847757,-4.07221045142267,
17.8653382206309));
#34993=CARTESIAN_POINT('Ctrl Pts',(3.22586952699263,-2.51287987232251,18.0642711589944));
#34994=CARTESIAN_POINT('Ctrl Pts',(3.85753348743574,1.35655256116935,18.2632040973578));
#34995=CARTESIAN_POINT('Ctrl Pts',(0.942949431467649,3.97890007760914,18.4621370357212));
#34996=CARTESIAN_POINT('Ctrl Pts',(-2.83849231006808,2.94342672128722,18.6610699740847));
#34997=CARTESIAN_POINT('Ctrl Pts',(-4.01049520759558,-0.797952158814143,
18.8600029124481));
#34998=CARTESIAN_POINT('Ctrl Pts',(-1.49563168618331,-3.80577000319091,
19.0589358508116));
#34999=CARTESIAN_POINT('Ctrl Pts',(2.3941728221794,-3.31492623680237,19.257868789175));
#35000=CARTESIAN_POINT('Ctrl Pts',(4.08300340529871,0.223344241524889,19.4568017275385));
#35001=CARTESIAN_POINT('Ctrl Pts',(2.01831045474011,3.55629334647608,19.6557346659019));
#35002=CARTESIAN_POINT('Ctrl Pts',(-1.90182444335736,3.61992586174797,19.8546676042653));
#35003=CARTESIAN_POINT('Ctrl Pts',(-4.07360351206664,0.355744127683883,
20.0536005426287));
#35004=CARTESIAN_POINT('Ctrl Pts',(-2.5005004115443,-3.23547479510659,20.2525334809922));
#35005=CARTESIAN_POINT('Ctrl Pts',(1.37132404897559,-3.85230707636404,20.4514664193556));
#35006=CARTESIAN_POINT('Ctrl Pts',(3.98248409676232,-0.927696004593339,
20.6503993577191));
#35007=CARTESIAN_POINT('Ctrl Pts',(2.93252846673791,2.84975020829459,20.8493322960825));
#35008=CARTESIAN_POINT('Ctrl Pts',(-0.813313872270502,4.00740814031659,
21.0482652344459));
#35009=CARTESIAN_POINT('Ctrl Pts',(-3.8114730827583,1.48103760833823,21.2471981728094));
#35010=CARTESIAN_POINT('Ctrl Pts',(-3.30572781558952,-2.40685750869074,
21.4461311111728));
#35011=CARTESIAN_POINT('Ctrl Pts',(0.238988013211991,-4.0821176106825,21.6450640495362));
#35012=CARTESIAN_POINT('Ctrl Pts',(3.56400107843168,-2.00466849400123,21.8439969878997));
#35013=CARTESIAN_POINT('Ctrl Pts',(3.61261180105568,1.91568145388957,22.0429299262631));
#35014=CARTESIAN_POINT('Ctrl Pts',(0.340132123483712,4.0749367598133,22.2418628646266));
#35015=CARTESIAN_POINT('Ctrl Pts',(-3.24503255660361,2.48808423580994,22.44079580299));
#35016=CARTESIAN_POINT('Ctrl Pts',(-3.84702410170021,-1.38607540157123,
22.6397287413534));
#35017=CARTESIAN_POINT('Ctrl Pts',(-0.912428956318338,-3.98600964092851,
22.8386616797169));
#35018=CARTESIAN_POINT('Ctrl Pts',(2.86096626351498,-2.92158715374577,23.0375946180803));
#35019=CARTESIAN_POINT('Ctrl Pts',(4.00426223208981,0.828663643803887,23.2365275564438));
#35020=CARTESIAN_POINT('Ctrl Pts',(1.46642178435367,3.81712019830084,23.4354604948072));
#35021=CARTESIAN_POINT('Ctrl Pts',(-2.4195068552087,3.29648085623159,23.6343934331707));
#35022=CARTESIAN_POINT('Ctrl Pts',(-4.08117187815611,-0.254628275827654,
23.8333263715341));
#35023=CARTESIAN_POINT('Ctrl Pts',(-1.99099709862783,-3.57165648000459,
24.0322593098975));
#35024=CARTESIAN_POINT('Ctrl Pts',(1.92951033638773,-3.60524469622744,24.2311922482609));
#35025=CARTESIAN_POINT('Ctrl Pts',(4.07621017508652,-0.324515125108852,
24.4301251866244));
#35026=CARTESIAN_POINT('Ctrl Pts',(2.47563152742672,3.2545426711466,24.6290581249878));
#35027=CARTESIAN_POINT('Ctrl Pts',(-1.40080640236154,3.84168464101443,24.8279910633513));
#35028=CARTESIAN_POINT('Ctrl Pts',(-3.98947665834203,0.897148510809323,
25.0269240017147));
#35029=CARTESIAN_POINT('Ctrl Pts',(-2.91060294296254,-2.8721403110435,25.2258569400782));
#35030=CARTESIAN_POINT('Ctrl Pts',(0.844001248033056,-4.00105752910675,
25.4247898784416));
#35031=CARTESIAN_POINT('Ctrl Pts',(3.82271126690174,-1.45178442883431,25.623722816805));
#35032=CARTESIAN_POINT('Ctrl Pts',(3.28718549450203,2.43212067600246,25.8226557551684));
#35033=CARTESIAN_POINT('Ctrl Pts',(-0.270264799725342,4.08016622160577,
26.0215886935319));
#35034=CARTESIAN_POINT('Ctrl Pts',(-3.57925943879032,1.97729646935751,26.2205216318953));
#35035=CARTESIAN_POINT('Ctrl Pts',(-3.59782465543471,-1.94331088780188,
26.4194545702588));
#35036=CARTESIAN_POINT('Ctrl Pts',(-0.308893361864258,-4.07742373918868,
26.6183875086222));
#35037=CARTESIAN_POINT('Ctrl Pts',(3.26400499909824,-2.46314246923822,26.8173204469857));
#35038=CARTESIAN_POINT('Ctrl Pts',(3.83628877270618,1.41551683505063,27.016253385349));
#35039=CARTESIAN_POINT('Ctrl Pts',(0.881854892429735,3.99288509809649,27.2151863237125));
#35040=CARTESIAN_POINT('Ctrl Pts',(-2.88327218681108,2.89957599566987,27.4141192620759));
#35041=CARTESIAN_POINT('Ctrl Pts',(-3.99779407842222,-0.859326459755243,
27.6130522004394));
#35042=CARTESIAN_POINT('Ctrl Pts',(-1.43712575670111,-3.82824620646707,
27.8119851388028));
#35043=CARTESIAN_POINT('Ctrl Pts',(2.44469878586269,-3.2778418668851,28.0109180771663));
#35044=CARTESIAN_POINT('Ctrl Pts',(4.07910065579756,0.285897355313241,28.2098510155297));
#35045=CARTESIAN_POINT('Ctrl Pts',(1.96356680735725,3.58680984315424,28.4087839538932));
#35046=CARTESIAN_POINT('Ctrl Pts',(-1.95708290549785,3.59035178762629,28.6077168922566));
#35047=CARTESIAN_POINT('Ctrl Pts',(-4.07857743430098,0.293267063125026,
28.80664983062));
#35048=CARTESIAN_POINT('Ctrl Pts',(-2.45061724462188,-3.27341940152267,
29.0055827689835));
#35049=CARTESIAN_POINT('Ctrl Pts',(1.43020648364449,-3.83083657600328,29.2045157073469));
#35050=CARTESIAN_POINT('Ctrl Pts',(3.99623491014561,-0.866548325736514,
29.4034486457103));
#35051=CARTESIAN_POINT('Ctrl Pts',(2.88850647377694,2.89436172736787,29.6023815840738));
#35052=CARTESIAN_POINT('Ctrl Pts',(-0.874639053949637,3.9944719279536,29.8013145224372));
#35053=CARTESIAN_POINT('Ctrl Pts',(-3.83372493572705,1.42244598318807,30.0002474608007));
#35054=CARTESIAN_POINT('Ctrl Pts',(-3.26845011057368,-2.45724100010441,
30.1991803991641));
#35055=CARTESIAN_POINT('Ctrl Pts',(0.301525713057809,-4.07797519637728,
30.3981133375275));
#35056=CARTESIAN_POINT('Ctrl Pts',(3.59430758223343,-1.94980831422029,30.5970462758909));
#35057=CARTESIAN_POINT('Ctrl Pts',(3.58282620252664,1.97082618726046,30.7959792142544));
#35058=CARTESIAN_POINT('Ctrl Pts',(0.277636458332829,4.07967124348368,30.9949121526178));
#35059=CARTESIAN_POINT('Ctrl Pts',(-3.2827857401879,2.4380560374861,31.1938450909813));
#35060=CARTESIAN_POINT('Ctrl Pts',(-3.82532813096051,-1.44487513245452,
31.3927780293447));
#35061=CARTESIAN_POINT('Ctrl Pts',(-0.851229035476529,-3.99952604530396,
31.5917109677081));
#35062=CARTESIAN_POINT('Ctrl Pts',(2.90540876988572,-2.877394539818,31.7906439060716));
#35063=CARTESIAN_POINT('Ctrl Pts',(3.99109112648016,0.889938805780879,31.989576844435));
#35064=CARTESIAN_POINT('Ctrl Pts',(1.4077453238388,3.83914737423731,32.1885097827985));
#35065=CARTESIAN_POINT('Ctrl Pts',(-2.46974713456985,3.25901036346728,32.3874427211619));
#35066=CARTESIAN_POINT('Ctrl Pts',(-4.07678985987002,-0.317149643487198,
32.5863756595253));
#35067=CARTESIAN_POINT('Ctrl Pts',(-1.93602119196322,-3.60175254593826,
32.7853085978888));
#35068=CARTESIAN_POINT('Ctrl Pts',(1.98454053129662,-3.57524801063428,32.9842415362522));
#35069=CARTESIAN_POINT('Ctrl Pts',(4.08070515067628,-0.262001776992349,
33.1831744746156));
#35070=CARTESIAN_POINT('Ctrl Pts',(2.42545903226761,3.29210387756742,33.3821074129791));
#35071=CARTESIAN_POINT('Ctrl Pts',(-1.45952256610013,3.81976351845869,33.5810403513425));
#35072=CARTESIAN_POINT('Ctrl Pts',(-4.00275845524774,0.835897246583656,
33.7799732897059));
#35073=CARTESIAN_POINT('Ctrl Pts',(-2.86624035694998,-2.91641315216041,
33.9789062280695));
#35074=CARTESIAN_POINT('Ctrl Pts',(0.905225490601913,-3.98765172364236,
34.1778391664328));
#35075=CARTESIAN_POINT('Ctrl Pts',(3.84451344237989,-1.3930239945038,34.3767721047963));
#35076=CARTESIAN_POINT('Ctrl Pts',(3.24952276417025,2.48221700563069,34.5757050431597));
#35077=CARTESIAN_POINT('Ctrl Pts',(-0.332768917194808,4.07554466368054,
34.7746379815232));
#35078=CARTESIAN_POINT('Ctrl Pts',(-3.60914462495387,1.92220564302213,34.9735709198866));
#35079=CARTESIAN_POINT('Ctrl Pts',(-3.56761732322031,-1.99822573623664,
35.17250385825));
#35080=CARTESIAN_POINT('Ctrl Pts',(-0.246363248667963,-4.08167914070044,
35.3714367966135));
#35081=CARTESIAN_POINT('Ctrl Pts',(3.30137367684192,-2.41282641392402,35.5703697349769));
#35082=CARTESIAN_POINT('Ctrl Pts',(3.81414282020493,1.47414856950349,35.7693026733403));
#35083=CARTESIAN_POINT('Ctrl Pts',(0.820553184171816,4.00593209253256,35.9682356117038));
#35084=CARTESIAN_POINT('Ctrl Pts',(-2.9273747126076,2.8550440889171,36.1671685500672));
#35085=CARTESIAN_POINT('Ctrl Pts',(-3.98415376995365,-0.920498883894049,
36.3661014884307));
#35086=CARTESIAN_POINT('Ctrl Pts',(-1.37828221131289,-3.849823061487,36.5650344267941));
#35087=CARTESIAN_POINT('Ctrl Pts',(2.49465043014533,-3.23998745175455,36.7639673651575));
#35088=CARTESIAN_POINT('Ctrl Pts',(4.07423962618006,0.348383304391666,36.962900303521));
#35089=CARTESIAN_POINT('Ctrl Pts',(1.90836187008279,3.61648371160565,37.1618332418844));
#35090=CARTESIAN_POINT('Ctrl Pts',(-2.01188160081678,3.55993425067045,37.3607661802478));
#35091=CARTESIAN_POINT('Ctrl Pts',(-4.08259319987495,0.230721106156537,
37.5596991186113));
#35092=CARTESIAN_POINT('Ctrl Pts',(-2.40015836675168,-3.31059500799247,
37.7586320569747));
#35093=CARTESIAN_POINT('Ctrl Pts',(1.48875292563011,-3.8084661070492,37.9575649953382));
#35094=CARTESIAN_POINT('Ctrl Pts',(4.00904691493279,-0.805197095935613,
38.1564979337016));
#35095=CARTESIAN_POINT('Ctrl Pts',(2.84380589172842,2.93829333322945,38.3554308720651));
#35096=CARTESIAN_POINT('Ctrl Pts',(-0.935758745314963,3.9805972344063,38.5543638104285));
#35097=CARTESIAN_POINT('Ctrl Pts',(-3.85507618443849,1.3635203486794,38.7532967487919));
#35098=CARTESIAN_POINT('Ctrl Pts',(-3.23040450708304,-2.50704752847379,
38.9522296871554));
#35099=CARTESIAN_POINT('Ctrl Pts',(0.363992462388689,-4.07287418561517,
39.1511626255188));
#35100=CARTESIAN_POINT('Ctrl Pts',(3.62376991564507,-1.8944911904441,39.3500955638822));
#35101=CARTESIAN_POINT('Ctrl Pts',(3.55219848867015,2.02551006091971,39.5490285022457));
#35102=CARTESIAN_POINT('Ctrl Pts',(0.215076379060282,4.08344321778653,39.7479614406091));
#35103=CARTESIAN_POINT('Ctrl Pts',(-3.31976926965591,2.38746293362043,39.9468943789726));
#35104=CARTESIAN_POINT('Ctrl Pts',(-3.80273052050235,-1.50335048727303,
40.145827317336));
#35105=CARTESIAN_POINT('Ctrl Pts',(-0.789834848961668,-4.01207398204883,
40.3447602556994));
#35106=CARTESIAN_POINT('Ctrl Pts',(2.94917967271135,-2.83258134221006,40.5436931940629));
#35107=CARTESIAN_POINT('Ctrl Pts',(3.97696142147388,0.951111115579423,40.7426261324263));
#35108=CARTESIAN_POINT('Ctrl Pts',(1.34877841142462,3.86006894220613,40.9415590707897));
#35109=CARTESIAN_POINT('Ctrl Pts',(-2.51948441896513,3.22116494326784,41.1404920091532));
#35110=CARTESIAN_POINT('Ctrl Pts',(-4.07130205620617,-0.380346269017061,
41.3394249475166));
#35111=CARTESIAN_POINT('Ctrl Pts',(-1.88087422963442,-3.62955985044473,
41.5383578858801));
#35112=CARTESIAN_POINT('Ctrl Pts',(2.0396473123645,-3.54722160642478,41.7372908242435));
#35113=CARTESIAN_POINT('Ctrl Pts',(4.08365574488659,-0.19291304504628,41.9362669284183));
#35114=CARTESIAN_POINT('Ctrl Pts',(2.94480488286648,2.14655679302897,42.0689320531386));
#35115=CARTESIAN_POINT('Ctrl Pts',(2.00570496136574,2.81548347365039,42.1352861984045));
#35116=CARTESIAN_POINT('Ctrl Pts',(1.6435788288222,-3.31109949314964,6.86350499875044));
#35117=CARTESIAN_POINT('Ctrl Pts',(2.74721907371341,-2.76326946119434,6.92981597820492));
#35118=CARTESIAN_POINT('Ctrl Pts',(4.34414919481839,-0.486393044209725,
7.06243793711388));
#35119=CARTESIAN_POINT('Ctrl Pts',(2.75379312724547,3.40034806728253,7.26137087547732));
#35120=CARTESIAN_POINT('Ctrl Pts',(-1.37188000734597,4.15061578131742,7.46030381384076));
#35121=CARTESIAN_POINT('Ctrl Pts',(-4.23445827724675,1.09043987287385,7.65923675220419));
#35122=CARTESIAN_POINT('Ctrl Pts',(-3.2052772200551,-2.97488551610267,7.85816969056764));
#35123=CARTESIAN_POINT('Ctrl Pts',(0.771049403037938,-4.30397858890673,
8.05710262893107));
#35124=CARTESIAN_POINT('Ctrl Pts',(4.03827586239305,-1.67713777828685,8.25603556729451));
#35125=CARTESIAN_POINT('Ctrl Pts',(3.59323830599447,2.49188565388108,8.45496850565795));
#35126=CARTESIAN_POINT('Ctrl Pts',(-0.155153181914435,4.36990798398716,
8.65390144402138));
#35127=CARTESIAN_POINT('Ctrl Pts',(-3.76087322949614,2.23075804087219,8.85283438238483));
#35128=CARTESIAN_POINT('Ctrl Pts',(-3.90922550655774,-1.95919207824947,
9.05176732074826));
#35129=CARTESIAN_POINT('Ctrl Pts',(-0.463798613632033,-4.34801977857419,
9.2507002591117));
#35130=CARTESIAN_POINT('Ctrl Pts',(3.40799499944848,-2.73970792995919,9.44963319747514));
#35131=CARTESIAN_POINT('Ctrl Pts',(4.14680620577778,1.38723751938316,9.64856613583857));
#35132=CARTESIAN_POINT('Ctrl Pts',(1.07343819364456,4.23888522314733,9.84749907420202));
#35133=CARTESIAN_POINT('Ctrl Pts',(-2.9867456421098,3.19370862133198,10.0464320125655));
#35134=CARTESIAN_POINT('Ctrl Pts',(-4.30120107661137,-0.787459878855247,
10.2453649509289));
#35135=CARTESIAN_POINT('Ctrl Pts',(-1.66154265936265,-4.04471237562304,
10.4442978892923));
#35136=CARTESIAN_POINT('Ctrl Pts',(2.50557934483546,-3.58364275211452,10.6432308276558));
#35137=CARTESIAN_POINT('Ctrl Pts',(4.36931095975112,0.171886048121829,10.8421637660192));
#35138=CARTESIAN_POINT('Ctrl Pts',(2.21631517892575,3.76939914480685,11.0410967043827));
#35139=CARTESIAN_POINT('Ctrl Pts',(-1.97414917416402,3.90168656767488,11.2400296427461));
#35140=CARTESIAN_POINT('Ctrl Pts',(-4.34976925317394,0.447135825469514,
11.4389625811095));
#35141=CARTESIAN_POINT('Ctrl Pts',(-2.72662674141349,-3.41846889597808,
11.6378955194729));
#35142=CARTESIAN_POINT('Ctrl Pts',(1.40311608794153,-4.14145967563326,11.8368284578364));
#35143=CARTESIAN_POINT('Ctrl Pts',(4.24296794021624,-1.057187804276,12.0357613961998));
#35144=CARTESIAN_POINT('Ctrl Pts',(3.18224013634397,2.99896160485262,12.2346943345633));
#35145=CARTESIAN_POINT('Ctrl Pts',(-0.803935445702029,4.29815202091405,
12.4336272729267));
#35146=CARTESIAN_POINT('Ctrl Pts',(-4.05104952943537,1.64603180552031,12.6325602112902));
#35147=CARTESIAN_POINT('Ctrl Pts',(-3.57401542229434,-2.51929290787779,
12.8314931496536));
#35148=CARTESIAN_POINT('Ctrl Pts',(0.18862725909364,-4.36862023435567,13.030426088017));
#35149=CARTESIAN_POINT('Ctrl Pts',(3.77786404640665,-2.20185518179452,13.2293590263804));
#35150=CARTESIAN_POINT('Ctrl Pts',(3.89409329547718,1.98908531763447,13.4282919647439));
#35151=CARTESIAN_POINT('Ctrl Pts',(0.430464930930045,4.35145067052408,13.6272249031073));
#35152=CARTESIAN_POINT('Ctrl Pts',(-3.42889179538761,2.71350770226696,13.8261578414708));
#35153=CARTESIAN_POINT('Ctrl Pts',(-4.13605275529299,-1.4189751936421,14.0250907798342));
#35154=CARTESIAN_POINT('Ctrl Pts',(-1.04092167366474,-4.246987763585,14.2240237181976));
#35155=CARTESIAN_POINT('Ctrl Pts',(3.01113341976998,-3.17072523613856,14.4229566565611));
#35156=CARTESIAN_POINT('Ctrl Pts',(4.29503991467939,0.820399369851541,14.6218895949245));
#35157=CARTESIAN_POINT('Ctrl Pts',(1.63049675193903,4.05732711728536,14.820822533288));
#35158=CARTESIAN_POINT('Ctrl Pts',(-2.53296946387702,3.56433565897051,15.0197554716514));
#35159=CARTESIAN_POINT('Ctrl Pts',(-4.36786537274413,-0.205365723345486,
15.2186884100148));
#35160=CARTESIAN_POINT('Ctrl Pts',(-2.18736285033501,-3.7862734655221,15.4176213483783));
#35161=CARTESIAN_POINT('Ctrl Pts',(2.00399225298804,-3.88644285236594,15.6165542867417));
#35162=CARTESIAN_POINT('Ctrl Pts',(4.35306819652955,-0.41378771260799,15.8154872251052));
#35163=CARTESIAN_POINT('Ctrl Pts',(2.70034881994612,3.43926434653661,16.0144201634686));
#35164=CARTESIAN_POINT('Ctrl Pts',(-1.43481346414344,4.13058510599347,16.213353101832));
#35165=CARTESIAN_POINT('Ctrl Pts',(-4.25094522841732,1.02464025869492,16.4122860401955));
#35166=CARTESIAN_POINT('Ctrl Pts',(-3.15916377994851,-3.02326102184444,
16.6112189785589));
#35167=CARTESIAN_POINT('Ctrl Pts',(0.836851247995388,-4.29186474431231,
16.8101519169224));
#35168=CARTESIAN_POINT('Ctrl Pts',(4.06354513124908,-1.61493775763784,17.0090848552858));
#35169=CARTESIAN_POINT('Ctrl Pts',(3.55460356033887,2.54660882814157,17.2080177936493));
#35170=CARTESIAN_POINT('Ctrl Pts',(-0.222101172196999,4.36704637759334,
17.4069507320126));
#35171=CARTESIAN_POINT('Ctrl Pts',(-3.79462729062322,2.17283840172248,17.6058836703761));
#35172=CARTESIAN_POINT('Ctrl Pts',(-3.87873534444371,-2.0188697636315,17.8048166087395));
#35173=CARTESIAN_POINT('Ctrl Pts',(-0.397104418623892,-4.35462180624813,
18.003749547103));
#35174=CARTESIAN_POINT('Ctrl Pts',(3.44958639881833,-2.68715028828496,18.2026824854664));
#35175=CARTESIAN_POINT('Ctrl Pts',(4.12505680713318,1.45063066721568,18.4016154238299));
#35176=CARTESIAN_POINT('Ctrl Pts',(1.00834379888781,4.25484027643657,18.6005483621933));
#35177=CARTESIAN_POINT('Ctrl Pts',(-3.03534423324606,3.14755593761926,18.7994813005568));
#35178=CARTESIAN_POINT('Ctrl Pts',(-4.28862655630873,-0.853290838615923,
18.9984142389201));
#35179=CARTESIAN_POINT('Ctrl Pts',(-1.59935505113543,-4.06970348000317,
19.1973471772837));
#35180=CARTESIAN_POINT('Ctrl Pts',(2.56021080043808,-3.54481926930875,19.396280115647));
#35181=CARTESIAN_POINT('Ctrl Pts',(4.36616326091091,0.238833359927311,19.5952130540105));
#35182=CARTESIAN_POINT('Ctrl Pts',(2.15828204922935,3.802925399047,19.7941459923739));
#35183=CARTESIAN_POINT('Ctrl Pts',(-2.03371763112254,3.87097088488195,19.9930789307374));
#35184=CARTESIAN_POINT('Ctrl Pts',(-4.3561114768656,0.380415293938357,20.1920118691008));
#35185=CARTESIAN_POINT('Ctrl Pts',(-2.67391230107938,-3.45985780067314,
20.3909448074643));
#35186=CARTESIAN_POINT('Ctrl Pts',(1.46642657061485,-4.11946793988461,20.5898777458277));
#35187=CARTESIAN_POINT('Ctrl Pts',(4.25867285045125,-0.992032533524869,
20.7888106841911));
#35188=CARTESIAN_POINT('Ctrl Pts',(3.13590187958944,3.0473828765565,20.9877436225545));
#35189=CARTESIAN_POINT('Ctrl Pts',(-0.869717900330041,4.28532539821516,
21.186676560918));
#35190=CARTESIAN_POINT('Ctrl Pts',(-4.07580207312432,1.58374886123332,21.3856094992814));
#35191=CARTESIAN_POINT('Ctrl Pts',(-3.53498292954331,-2.57377518104822,
21.5845424376449));
#35192=CARTESIAN_POINT('Ctrl Pts',(0.255562040857054,-4.36521603566368,
21.7834753760083));
#35193=CARTESIAN_POINT('Ctrl Pts',(3.81116766895198,-2.14369400658712,21.9824083143717));
#35194=CARTESIAN_POINT('Ctrl Pts',(3.86314958768654,2.04853563744927,22.1813412527352));
#35195=CARTESIAN_POINT('Ctrl Pts',(0.363720583598531,4.35753718650904,22.3802741910986));
#35196=CARTESIAN_POINT('Ctrl Pts',(-3.47007840128558,2.66063505270333,22.5792071294621));
#35197=CARTESIAN_POINT('Ctrl Pts',(-4.11381858630935,-1.48220094240897,
22.7781400678255));
#35198=CARTESIAN_POINT('Ctrl Pts',(-0.975706702105193,-4.26244289418747,
22.9770730061889));
#35199=CARTESIAN_POINT('Ctrl Pts',(3.05937677501175,-3.12420177697617,23.1760059445524));
#35200=CARTESIAN_POINT('Ctrl Pts',(4.28196131850264,0.886132191938384,23.3749388829158));
#35201=CARTESIAN_POINT('Ctrl Pts',(1.56811941707795,4.08184082106659,23.5738718212792));
#35202=CARTESIAN_POINT('Ctrl Pts',(-2.58730177080555,3.52509468547,23.7728047596427));
#35203=CARTESIAN_POINT('Ctrl Pts',(-4.3642047157598,-0.272286969358187,
23.9717376980061));
#35204=CARTESIAN_POINT('Ctrl Pts',(-2.12907448799273,-3.81935397931651,
24.1706706363695));
#35205=CARTESIAN_POINT('Ctrl Pts',(2.06332356503822,-3.85527156769798,24.369603574733));
#35206=CARTESIAN_POINT('Ctrl Pts',(4.3588989142447,-0.347020532733638,24.5685365130964));
#35207=CARTESIAN_POINT('Ctrl Pts',(2.6473187381073,3.4802480505861,24.7674694514599));
#35208=CARTESIAN_POINT('Ctrl Pts',(-1.49795355098226,4.10810882935714,24.9664023898233));
#35209=CARTESIAN_POINT('Ctrl Pts',(-4.26615035228957,0.959366544341607,
25.1653353281867));
#35210=CARTESIAN_POINT('Ctrl Pts',(-3.11245580157246,-3.07132575250498,
25.3642682665502));
#35211=CARTESIAN_POINT('Ctrl Pts',(0.902533472429329,-4.27853436656609,
25.5632012049136));
#35212=CARTESIAN_POINT('Ctrl Pts',(4.0878196351628,-1.55246694815701,25.7621341432771));
#35213=CARTESIAN_POINT('Ctrl Pts',(3.51515468227829,2.60079037109864,25.9610670816405));
#35214=CARTESIAN_POINT('Ctrl Pts',(-0.289007899857984,4.36312931604853,
26.160000020004));
#35215=CARTESIAN_POINT('Ctrl Pts',(-3.8274842099407,2.11442370810511,26.3589329583674));
#35216=CARTESIAN_POINT('Ctrl Pts',(-3.8473369405895,-2.07808119675769,26.5578658967308));
#35217=CARTESIAN_POINT('Ctrl Pts',(-0.330315386551131,-4.36019664007829,
26.7567988350943));
#35218=CARTESIAN_POINT('Ctrl Pts',(3.49036659925336,-2.6339635528152,26.9557317734577));
#35219=CARTESIAN_POINT('Ctrl Pts',(4.10233875286451,1.51368416503854,27.1546647118211));
#35220=CARTESIAN_POINT('Ctrl Pts',(0.943012300157368,4.26979517032074,27.3535976501846));
#35221=CARTESIAN_POINT('Ctrl Pts',(-3.08322963358878,3.10066412584504,27.552530588548));
#35222=CARTESIAN_POINT('Ctrl Pts',(-4.27504459272359,-0.9189215009821,27.7514635269115));
#35223=CARTESIAN_POINT('Ctrl Pts',(-1.53679168429643,-4.09373842762575,
27.9503964652748));
#35224=CARTESIAN_POINT('Ctrl Pts',(2.61424078387375,-3.50516306591769,28.1493294036383));
#35225=CARTESIAN_POINT('Ctrl Pts',(4.36198985231999,0.305724586842239,28.3482623420017));
#35226=CARTESIAN_POINT('Ctrl Pts',(2.09974188204234,3.835558241448,28.5471952803652));
#35227=CARTESIAN_POINT('Ctrl Pts',(-2.09280831592068,3.83934582286561,28.7461282187286));
#35228=CARTESIAN_POINT('Ctrl Pts',(-4.36143034495521,0.313605390333471,
28.9450611570921));
#35229=CARTESIAN_POINT('Ctrl Pts',(-2.62056969292188,-3.50043389871622,
29.1439940954555));
#35230=CARTESIAN_POINT('Ctrl Pts',(1.52939255360441,-4.09650844155383,29.342927033819));
#35231=CARTESIAN_POINT('Ctrl Pts',(4.27337729476395,-0.926644209682624,
29.5418599721824));
#35232=CARTESIAN_POINT('Ctrl Pts',(3.08882692293162,3.09508824347791,29.7407929105458));
#35233=CARTESIAN_POINT('Ctrl Pts',(-0.935296036970499,4.27149204821567,
29.9397258489092));
#35234=CARTESIAN_POINT('Ctrl Pts',(-4.09959711154953,1.52109385565686,30.1386587872727));
#35235=CARTESIAN_POINT('Ctrl Pts',(-3.49511998309561,-2.62765281163783,
30.3375917256362));
#35236=CARTESIAN_POINT('Ctrl Pts',(0.322436784859063,-4.360786341305,30.5365246639996));
#35237=CARTESIAN_POINT('Ctrl Pts',(3.84357595528703,-2.08502922537836,30.735457602363));
#35238=CARTESIAN_POINT('Ctrl Pts',(3.83129833186026,2.10750470628822,30.9343905407264));
#35239=CARTESIAN_POINT('Ctrl Pts',(0.296890789434302,4.36260001076095,31.1333234790899));
#35240=CARTESIAN_POINT('Ctrl Pts',(-3.51044980115615,2.60713735508994,31.3322564174533));
#35241=CARTESIAN_POINT('Ctrl Pts',(-4.09061798103173,-1.54507848603308,
31.5311893558168));
#35242=CARTESIAN_POINT('Ctrl Pts',(-0.910262513250637,-4.27689667302272,
31.7301222941802));
#35243=CARTESIAN_POINT('Ctrl Pts',(3.10690140805196,-3.07694436663831,31.9290552325437));
#35244=CARTESIAN_POINT('Ctrl Pts',(4.26787678520448,0.951656839966625,32.127988170907));
#35245=CARTESIAN_POINT('Ctrl Pts',(1.50537369273006,4.10539560091092,32.3269211092706));
#35246=CARTESIAN_POINT('Ctrl Pts',(-2.64102625746159,3.48502558127492,32.5258540476339));
#35247=CARTESIAN_POINT('Ctrl Pts',(-4.35951880067472,-0.339144248522522,
32.7247869859974));
#35248=CARTESIAN_POINT('Ctrl Pts',(-2.07028595413972,-3.85153723373335,
32.9237199243608));
#35249=CARTESIAN_POINT('Ctrl Pts',(2.12217015207268,-3.82319458573513,33.1226528627243));
#35250=CARTESIAN_POINT('Ctrl Pts',(4.36370562032123,-0.280171829274663,
33.3215858010877));
#35251=CARTESIAN_POINT('Ctrl Pts',(2.59366673654697,3.52041415950907,33.5205187394511));
#35252=CARTESIAN_POINT('Ctrl Pts',(-1.56074173200713,4.08466745778821,33.7194516778146));
#35253=CARTESIAN_POINT('Ctrl Pts',(-4.28035325342194,0.893867451394637,
33.9183846161781));
#35254=CARTESIAN_POINT('Ctrl Pts',(-3.06501663143715,-3.11866895385767,
34.1173175545414));
#35255=CARTESIAN_POINT('Ctrl Pts',(0.968003669743968,-4.26419885677308,
34.3162504929049));
#35256=CARTESIAN_POINT('Ctrl Pts',(4.11113381057032,-1.48963142633595,34.5151834312683));
#35257=CARTESIAN_POINT('Ctrl Pts',(3.47488000867237,2.65436092498193,34.7141163696317));
#35258=CARTESIAN_POINT('Ctrl Pts',(-0.355846732516481,4.35818724904092,
34.9130493079952));
#35259=CARTESIAN_POINT('Ctrl Pts',(-3.85944195989102,2.05551228480171,35.1119822463586));
#35260=CARTESIAN_POINT('Ctrl Pts',(-3.81503470347808,-2.13680443793921,
35.3109151847221));
#35261=CARTESIAN_POINT('Ctrl Pts',(-0.263448755339423,-4.36474715740505,
35.5098481230855));
#35262=CARTESIAN_POINT('Ctrl Pts',(3.53032682746711,-2.58015803507752,35.708781061449));
#35263=CARTESIAN_POINT('Ctrl Pts',(4.07865695919681,1.5763820615329,35.9077139998124));
#35264=CARTESIAN_POINT('Ctrl Pts',(0.87745926484041,4.28374698522694,36.1066469381758));
#35265=CARTESIAN_POINT('Ctrl Pts',(-3.13039070810472,3.05304389242815,36.3055798765393));
#35266=CARTESIAN_POINT('Ctrl Pts',(-4.26045831693806,-0.984336286213261,
36.5045128149027));
#35267=CARTESIAN_POINT('Ctrl Pts',(-1.47386728759316,-4.11681165640429,
36.7034457532661));
#35268=CARTESIAN_POINT('Ctrl Pts',(2.66765661835625,-3.46468341400465,36.9023786916296));
#35269=CARTESIAN_POINT('Ctrl Pts',(4.35679170604889,0.372543991115891,37.101311629993));
#35270=CARTESIAN_POINT('Ctrl Pts',(2.04070843410648,3.86729001861809,37.3002445683564));
#35271=CARTESIAN_POINT('Ctrl Pts',(-2.15140734866625,3.80681880313016,37.4991775067199));
#35272=CARTESIAN_POINT('Ctrl Pts',(-4.3657246073824,0.246721816570115,37.6981104450834));
#35273=CARTESIAN_POINT('Ctrl Pts',(-2.56661144775907,-3.54018766599446,
37.8970433834468));
#35274=CARTESIAN_POINT('Ctrl Pts',(1.59199924252436,-4.07258656102101,38.0959763218102));
#35275=CARTESIAN_POINT('Ctrl Pts',(4.28707782328367,-0.861038218460384,
38.2949092601736));
#35276=CARTESIAN_POINT('Ctrl Pts',(3.04102631643975,3.14206654461201,38.4938421985371));
#35277=CARTESIAN_POINT('Ctrl Pts',(-1.00065443236423,4.25665513254129,38.6927751369005));
#35278=CARTESIAN_POINT('Ctrl Pts',(-4.12242908802487,1.45808167688089,38.8917080752639));
#35279=CARTESIAN_POINT('Ctrl Pts',(-3.45443588374254,-2.68091346629163,
39.0906410136274));
#35280=CARTESIAN_POINT('Ctrl Pts',(0.389235657865896,-4.35533157098711,
39.2895739519908));
#35281=CARTESIAN_POINT('Ctrl Pts',(3.8750815272774,-2.02587581070879,39.4885068903542));
#35282=CARTESIAN_POINT('Ctrl Pts',(3.79854655927238,2.16598095439164,39.6874398287178));
#35283=CARTESIAN_POINT('Ctrl Pts',(0.22999211397275,4.36663357477926,39.8863727670811));
#35284=CARTESIAN_POINT('Ctrl Pts',(-3.5499981707246,2.55303557524153,40.0853057054446));
#35285=CARTESIAN_POINT('Ctrl Pts',(-4.06645320653296,-1.60760915782874,
40.284238643808));
#35286=CARTESIAN_POINT('Ctrl Pts',(-0.844610586228765,-4.29031482015054,
40.4831715821715));
#35287=CARTESIAN_POINT('Ctrl Pts',(3.15370786125407,-3.02902333459953,40.6821045205349));
#35288=CARTESIAN_POINT('Ctrl Pts',(4.2527671728035,1.01707150292793,40.8810374588983));
#35289=CARTESIAN_POINT('Ctrl Pts',(1.44231737338975,4.12776809790848,41.0799703972618));
#35290=CARTESIAN_POINT('Ctrl Pts',(-2.69421286601115,3.44455554809932,41.2789033356252));
#35291=CARTESIAN_POINT('Ctrl Pts',(-4.3536504130292,-0.406723615280815,
41.4778362739886));
#35292=CARTESIAN_POINT('Ctrl Pts',(-2.0113145017627,-3.88127299911711,41.6767692123521));
#35293=CARTESIAN_POINT('Ctrl Pts',(2.18109863658322,-3.79322452589238,41.8757021507155));
#35294=CARTESIAN_POINT('Ctrl Pts',(4.3668608408195,-0.206291733369188,42.0746782548904));
#35295=CARTESIAN_POINT('Ctrl Pts',(3.14902967590887,2.29542238319448,42.2073433796106));
#35296=CARTESIAN_POINT('Ctrl Pts',(2.14480235386948,3.01073971390795,42.2736975248765));
#35297=CARTESIAN_POINT('Ctrl Pts',(1.75017024926294,-3.52583503975451,7.00191632522251));
#35298=CARTESIAN_POINT('Ctrl Pts',(2.92538514533336,-2.94247645252568,7.06822730467699));
#35299=CARTESIAN_POINT('Ctrl Pts',(4.62588136680913,-0.517937211465701,
7.20084926358595));
#35300=CARTESIAN_POINT('Ctrl Pts',(2.93238554756965,3.6208716735304,7.39978220194938));
#35301=CARTESIAN_POINT('Ctrl Pts',(-1.46085087755489,4.41979668342923,7.59871514031282));
#35302=CARTESIAN_POINT('Ctrl Pts',(-4.5090766372874,1.16115843709268,7.79764807867627));
#35303=CARTESIAN_POINT('Ctrl Pts',(-3.4131498488579,-3.16781649528616,7.99658101703969));
#35304=CARTESIAN_POINT('Ctrl Pts',(0.821054458870111,-4.58310556675101,
8.19551395540314));
#35305=CARTESIAN_POINT('Ctrl Pts',(4.30017115622109,-1.78590560549867,8.39444689376657));
#35306=CARTESIAN_POINT('Ctrl Pts',(3.82627147014904,2.65349252467134,8.59337983213001));
#35307=CARTESIAN_POINT('Ctrl Pts',(-0.165215369231643,4.65331069704242,
8.79231277049345));
#35308=CARTESIAN_POINT('Ctrl Pts',(-4.00477806241297,2.37542993860311,8.99124570885689));
#35309=CARTESIAN_POINT('Ctrl Pts',(-4.16275146604314,-2.0862520420764,9.19017864722033));
#35310=CARTESIAN_POINT('Ctrl Pts',(-0.493877458746418,-4.63000297048149,
9.38911158558376));
#35311=CARTESIAN_POINT('Ctrl Pts',(3.62901453406151,-2.91738687953307,9.5880445239472));
#35312=CARTESIAN_POINT('Ctrl Pts',(4.41574004455383,1.47720437408262,9.78697746231064));
#35313=CARTESIAN_POINT('Ctrl Pts',(1.14305414379514,4.513790684995,9.98591040067408));
#35314=CARTESIAN_POINT('Ctrl Pts',(-3.18044578895083,3.40083098896765,10.1848433390375));
#35315=CARTESIAN_POINT('Ctrl Pts',(-4.58014792377031,-0.838529207295953,
10.3837762774009));
#35316=CARTESIAN_POINT('Ctrl Pts',(-1.76929909250628,-4.30702509822045,
10.5827092157644));
#35317=CARTESIAN_POINT('Ctrl Pts',(2.66807429591995,-3.81605361346254,10.7816421541278));
#35318=CARTESIAN_POINT('Ctrl Pts',(4.65267495384734,0.183033416110524,10.9805750924913));
#35319=CARTESIAN_POINT('Ctrl Pts',(2.36005041019255,4.01385691099803,11.1795080308547));
#35320=CARTESIAN_POINT('Ctrl Pts',(-2.10217915419658,4.15472360250998,11.3784409692181));
#35321=CARTESIAN_POINT('Ctrl Pts',(-4.63186590418606,0.476134034701025,
11.5773739075816));
#35322=CARTESIAN_POINT('Ctrl Pts',(-2.90345733346189,-3.6401676967687,11.776306845945));
#35323=CARTESIAN_POINT('Ctrl Pts',(1.49411271933775,-4.41004677458003,11.9752397843084));
#35324=CARTESIAN_POINT('Ctrl Pts',(4.51813817951421,-1.12574986394373,12.1741727226719));
#35325=CARTESIAN_POINT('Ctrl Pts',(3.38861873551307,3.19345399651813,12.3731056610353));
#35326=CARTESIAN_POINT('Ctrl Pts',(-0.856073268115742,4.57690112691687,
12.5720385993988));
#35327=CARTESIAN_POINT('Ctrl Pts',(-4.3137732370215,1.75278230945974,12.7709715377622));
#35328=CARTESIAN_POINT('Ctrl Pts',(-3.80580192006295,-2.68267722802591,
12.9699044761256));
#35329=CARTESIAN_POINT('Ctrl Pts',(0.200860348938858,-4.6519394326686,13.1688374144891));
#35330=CARTESIAN_POINT('Ctrl Pts',(4.0228707889351,-2.34465263532486,13.3677703528525));
#35331=CARTESIAN_POINT('Ctrl Pts',(4.14663788197017,2.11808395503869,13.566703291216));
#35332=CARTESIAN_POINT('Ctrl Pts',(0.458381978553845,4.63365636690753,13.7656362295794));
#35333=CARTESIAN_POINT('Ctrl Pts',(-3.65126655502712,2.88948748205561,13.9645691679428));
#35334=CARTESIAN_POINT('Ctrl Pts',(-4.4042891979103,-1.51100033950559,14.1635021063063));
#35335=CARTESIAN_POINT('Ctrl Pts',(-1.10842882197895,-4.52241870147271,
14.3624350446697));
#35336=CARTESIAN_POINT('Ctrl Pts',(3.20641519313028,-3.37635705666365,14.5613679830331));
#35337=CARTESIAN_POINT('Ctrl Pts',(4.57358719049415,0.873604931171569,14.7603009213966));
#35338=CARTESIAN_POINT('Ctrl Pts',(1.73623975724267,4.32045794681424,14.95923385976));
#35339=CARTESIAN_POINT('Ctrl Pts',(-2.69724075306194,3.79549439267688,15.1581667981235));
#35340=CARTESIAN_POINT('Ctrl Pts',(-4.65113561583202,-0.218684356913533,
15.3570997364869));
#35341=CARTESIAN_POINT('Ctrl Pts',(-2.32922042914278,-4.03182558616862,
15.5560326748503));
#35342=CARTESIAN_POINT('Ctrl Pts',(2.13395765352274,-4.13849128279759,15.7549656132138));
#35343=CARTESIAN_POINT('Ctrl Pts',(4.63537879472331,-0.44062318850625,15.9538985515772));
#35344=CARTESIAN_POINT('Ctrl Pts',(2.87547520351587,3.66231179977693,16.1528314899406));
#35345=CARTESIAN_POINT('Ctrl Pts',(-1.52786577324392,4.39846695381126,16.3517644283041));
#35346=CARTESIAN_POINT('Ctrl Pts',(-4.52663282074132,1.09109150441536,16.5506973666675));
#35347=CARTESIAN_POINT('Ctrl Pts',(-3.36404580252289,-3.21932930955316,
16.749630305031));
#35348=CARTESIAN_POINT('Ctrl Pts',(0.891123766999176,-4.57020610002538,
16.9485632433944));
#35349=CARTESIAN_POINT('Ctrl Pts',(4.32707921916088,-1.71967171167232,17.1474961817578));
#35350=CARTESIAN_POINT('Ctrl Pts',(3.78513113586845,2.7117646743586,17.3464291201213));
#35351=CARTESIAN_POINT('Ctrl Pts',(-0.236505153929377,4.65026350618809,
17.5453620584847));
#35352=CARTESIAN_POINT('Ctrl Pts',(-4.0407211839356,2.31375402290608,17.7442949968481));
#35353=CARTESIAN_POINT('Ctrl Pts',(-4.13028391797584,-2.14980001900876,
17.9432279352116));
#35354=CARTESIAN_POINT('Ctrl Pts',(-0.422857928770215,-4.63703316107358,
18.142160873575));
#35355=CARTESIAN_POINT('Ctrl Pts',(3.67330327064404,-2.86142070424742,18.3410938119385));
#35356=CARTESIAN_POINT('Ctrl Pts',(4.39258012683063,1.544708773262,18.5400267503019));
#35357=CARTESIAN_POINT('Ctrl Pts',(1.07373816630795,4.53078047526401,18.7389596886653));
#35358=CARTESIAN_POINT('Ctrl Pts',(-3.23219615642406,3.35168515395129,18.9378926270288));
#35359=CARTESIAN_POINT('Ctrl Pts',(-4.56675790502189,-0.9086295184177,19.1368255653922));
#35360=CARTESIAN_POINT('Ctrl Pts',(-1.70307841608756,-4.33363695681545,
19.3357585037557));
#35361=CARTESIAN_POINT('Ctrl Pts',(2.72624877869676,-3.77471230181512,19.5346914421191));
#35362=CARTESIAN_POINT('Ctrl Pts',(4.6493231165231,0.254322478329726,19.7336243804825));
#35363=CARTESIAN_POINT('Ctrl Pts',(2.2982536437186,4.04955745161791,19.932557318846));
#35364=CARTESIAN_POINT('Ctrl Pts',(-2.16561081888772,4.12201590801593,20.1314902572094));
#35365=CARTESIAN_POINT('Ctrl Pts',(-4.63861944166455,0.405086460192834,
20.3304231955728));
#35366=CARTESIAN_POINT('Ctrl Pts',(-2.84732419061446,-3.68424080623969,
20.5293561339363));
#35367=CARTESIAN_POINT('Ctrl Pts',(1.56152909225411,-4.38662880340519,20.7282890722997));
#35368=CARTESIAN_POINT('Ctrl Pts',(4.53486160414019,-1.05636906245639,20.9272220106632));
#35369=CARTESIAN_POINT('Ctrl Pts',(3.33927529244099,3.24501554481841,21.1261549490266));
#35370=CARTESIAN_POINT('Ctrl Pts',(-0.926121928389577,4.56324265611374,
21.32508788739));
#35371=CARTESIAN_POINT('Ctrl Pts',(-4.34013106349035,1.68646011412841,21.5240208257534));
#35372=CARTESIAN_POINT('Ctrl Pts',(-3.76423804349709,-2.74069285340571,
21.7229537641169));
#35373=CARTESIAN_POINT('Ctrl Pts',(0.272136068502114,-4.64831446064486,
21.9218867024803));
#35374=CARTESIAN_POINT('Ctrl Pts',(4.05833425947229,-2.282719519173,22.1208196408438));
#35375=CARTESIAN_POINT('Ctrl Pts',(4.1136873743174,2.18138982100898,22.3197525792072));
#35376=CARTESIAN_POINT('Ctrl Pts',(0.387309043713353,4.64013761320478,22.5186855175706));
#35377=CARTESIAN_POINT('Ctrl Pts',(-3.69512424596756,2.83318586959673,22.7176184559341));
#35378=CARTESIAN_POINT('Ctrl Pts',(-4.38061307091849,-1.5783264832467,22.9165513942975));
#35379=CARTESIAN_POINT('Ctrl Pts',(-1.03898444789204,-4.53887614744645,
23.115484332661));
#35380=CARTESIAN_POINT('Ctrl Pts',(3.25778728650852,-3.32681640020656,23.3144172710244));
#35381=CARTESIAN_POINT('Ctrl Pts',(4.55966040491547,0.943600740072882,23.5133502093879));
#35382=CARTESIAN_POINT('Ctrl Pts',(1.66981704980222,4.34656144383233,23.7122831477513));
#35383=CARTESIAN_POINT('Ctrl Pts',(-2.7550966864024,3.75370851470842,23.9112160861147));
#35384=CARTESIAN_POINT('Ctrl Pts',(-4.6472375533635,-0.289945662888717,
24.1101490244782));
#35385=CARTESIAN_POINT('Ctrl Pts',(-2.26715187735763,-4.06705147862843,
24.3090819628416));
#35386=CARTESIAN_POINT('Ctrl Pts',(2.19713679368869,-4.10529843916849,24.508014901205));
#35387=CARTESIAN_POINT('Ctrl Pts',(4.6415876534029,-0.369525940358427,24.7069478395685));
#35388=CARTESIAN_POINT('Ctrl Pts',(2.81900594878788,3.70595343002559,24.9058807779319));
#35389=CARTESIAN_POINT('Ctrl Pts',(-1.59510069960298,4.37453301769984,25.1048137162954));
#35390=CARTESIAN_POINT('Ctrl Pts',(-4.54282404623711,1.02158457787389,25.3037466546588));
#35391=CARTESIAN_POINT('Ctrl Pts',(-3.31430866018239,-3.27051119396646,
25.5026795930222));
#35392=CARTESIAN_POINT('Ctrl Pts',(0.961065696825607,-4.55601120402541,
25.7016125313856));
#35393=CARTESIAN_POINT('Ctrl Pts',(4.35292800342385,-1.65314946747969,25.9005454697491));
#35394=CARTESIAN_POINT('Ctrl Pts',(3.74312387005455,2.76946006619482,26.0994784081125));
#35395=CARTESIAN_POINT('Ctrl Pts',(-0.307750999990631,4.64609241049128,
26.298411346476));
#35396=CARTESIAN_POINT('Ctrl Pts',(-4.0757089810911,2.25155094685271,26.4973442848394));
#35397=CARTESIAN_POINT('Ctrl Pts',(-4.09684922574428,-2.21285150571349,
26.6962772232029));
#35398=CARTESIAN_POINT('Ctrl Pts',(-0.351737411238005,-4.64296954096788,
26.8952101615663));
#35399=CARTESIAN_POINT('Ctrl Pts',(3.71672819940849,-2.8047846363922,27.0941430999298));
#35400=CARTESIAN_POINT('Ctrl Pts',(4.36838873302285,1.61185149502644,27.2930760382932));
#35401=CARTESIAN_POINT('Ctrl Pts',(1.00416970788501,4.54670524254498,27.4920089766566));
#35402=CARTESIAN_POINT('Ctrl Pts',(-3.28318708036648,3.30175225602021,27.69094191502));
#35403=CARTESIAN_POINT('Ctrl Pts',(-4.55229510702496,-0.97851654220896,
27.8898748533835));
#35404=CARTESIAN_POINT('Ctrl Pts',(-1.63645761189174,-4.35923064878442,
28.0888077917469));
#35405=CARTESIAN_POINT('Ctrl Pts',(2.78378278188482,-3.7324842649503,28.2877407301104));
#35406=CARTESIAN_POINT('Ctrl Pts',(4.6448790488424,0.32555181837124,28.4866736684738));
#35407=CARTESIAN_POINT('Ctrl Pts',(2.23591695672744,4.08430663974176,28.6856066068372));
#35408=CARTESIAN_POINT('Ctrl Pts',(-2.22853372634353,4.08833985810493,28.8845395452007));
#35409=CARTESIAN_POINT('Ctrl Pts',(-4.64428325560944,0.333943717541912,
29.0834724835641));
#35410=CARTESIAN_POINT('Ctrl Pts',(-2.79052214122188,-3.72744839590976,
29.2824054219276));
#35411=CARTESIAN_POINT('Ctrl Pts',(1.62857862356433,-4.36218030710437,29.481338360291));
#35412=CARTESIAN_POINT('Ctrl Pts',(4.55051967938229,-0.986740093628734,
29.6802712986544));
#35413=CARTESIAN_POINT('Ctrl Pts',(3.28914737208629,3.29581475958795,29.8792042370179));
#35414=CARTESIAN_POINT('Ctrl Pts',(-0.995953019991353,4.54851216847773,
30.0781371753813));
#35415=CARTESIAN_POINT('Ctrl Pts',(-4.36546928737203,1.61974172812565,30.2770701137447));
#35416=CARTESIAN_POINT('Ctrl Pts',(-3.72178985561752,-2.79806462317125,
30.4760030521082));
#35417=CARTESIAN_POINT('Ctrl Pts',(0.343347856660311,-4.64359748623272,
30.6749359904716));
#35418=CARTESIAN_POINT('Ctrl Pts',(4.09284432834063,-2.22025013653641,30.8738689288351));
#35419=CARTESIAN_POINT('Ctrl Pts',(4.07977046119387,2.24418322531598,31.0728018671985));
#35420=CARTESIAN_POINT('Ctrl Pts',(0.316145120535775,4.64552877803824,31.2717348055619));
#35421=CARTESIAN_POINT('Ctrl Pts',(-3.73811386212439,2.77621867269378,31.4706677439254));
#35422=CARTESIAN_POINT('Ctrl Pts',(-4.35590783110296,-1.64528183961164,
31.6696006822888));
#35423=CARTESIAN_POINT('Ctrl Pts',(-0.969295991024743,-4.55426730074148,
31.8685336206522));
#35424=CARTESIAN_POINT('Ctrl Pts',(3.30839404621819,-3.27649419345861,32.0674665590156));
#35425=CARTESIAN_POINT('Ctrl Pts',(4.54466244392879,1.01337487415237,32.2663994973791));
#35426=CARTESIAN_POINT('Ctrl Pts',(1.60300206162132,4.3716438275845,32.4653324357425));
#35427=CARTESIAN_POINT('Ctrl Pts',(-2.81230538035333,3.71104079908257,32.664265374106));
#35428=CARTESIAN_POINT('Ctrl Pts',(-4.64224774147941,-0.361138853557849,
32.8631983124694));
#35429=CARTESIAN_POINT('Ctrl Pts',(-2.20455071631624,-4.10132192152844,
33.0621312508329));
#35430=CARTESIAN_POINT('Ctrl Pts',(2.25979977284874,-4.07114116083598,33.2610641891963));
#35431=CARTESIAN_POINT('Ctrl Pts',(4.64670608996618,-0.298341881556976,
33.4599971275598));
#35432=CARTESIAN_POINT('Ctrl Pts',(2.76187444082632,3.74872444145071,33.6589300659231));
#35433=CARTESIAN_POINT('Ctrl Pts',(-1.66196089791414,4.34957139711773,33.8578630042867));
#35434=CARTESIAN_POINT('Ctrl Pts',(-4.55794805159614,0.951837656205623,
34.05679594265));
#35435=CARTESIAN_POINT('Ctrl Pts',(-3.26379290592433,-3.32092475555494,
34.2557288810135));
#35436=CARTESIAN_POINT('Ctrl Pts',(1.03078184888602,-4.54074598990379,34.4546618193769));
#35437=CARTESIAN_POINT('Ctrl Pts',(4.37775417876074,-1.58623885816811,34.6535947577404));
#35438=CARTESIAN_POINT('Ctrl Pts',(3.70023725317449,2.82650484433319,34.8525276961038));
#35439=CARTESIAN_POINT('Ctrl Pts',(-0.378924547838154,4.64082983440129,
35.0514606344673));
#35440=CARTESIAN_POINT('Ctrl Pts',(-4.10973929482816,2.18881892658129,35.2503935728307));
#35441=CARTESIAN_POINT('Ctrl Pts',(-4.06245208373585,-2.27538313964179,
35.4493265111941));
#35442=CARTESIAN_POINT('Ctrl Pts',(-0.280534262010886,-4.64781517410965,
35.6482594495575));
#35443=CARTESIAN_POINT('Ctrl Pts',(3.75927997809232,-2.74748965623102,35.847192387921));
#35444=CARTESIAN_POINT('Ctrl Pts',(4.34317109818868,1.67861555356232,36.0461253262844));
#35445=CARTESIAN_POINT('Ctrl Pts',(0.934365345509009,4.56156187792131,36.2450582646479));
#35446=CARTESIAN_POINT('Ctrl Pts',(-3.33340670360185,3.25104369593922,36.4439912030113));
#35447=CARTESIAN_POINT('Ctrl Pts',(-4.53676286392246,-1.04817368853247,
36.6429241413748));
#35448=CARTESIAN_POINT('Ctrl Pts',(-1.56945236387344,-4.38380025132158,
36.8418570797382));
#35449=CARTESIAN_POINT('Ctrl Pts',(2.84066280656719,-3.68937937625476,37.0407900181016));
#35450=CARTESIAN_POINT('Ctrl Pts',(4.63934378591771,0.396704677840125,37.239722956465));
#35451=CARTESIAN_POINT('Ctrl Pts',(2.17305499813018,4.11809632563053,37.4386558948285));
#35452=CARTESIAN_POINT('Ctrl Pts',(-2.29093309651572,4.05370335558988,37.6375888331919));
#35453=CARTESIAN_POINT('Ctrl Pts',(-4.64885601488985,0.262722526983691,
37.8365217715554));
#35454=CARTESIAN_POINT('Ctrl Pts',(-2.73306452876649,-3.76978032399644,
38.0354547099188));
#35455=CARTESIAN_POINT('Ctrl Pts',(1.69524555941862,-4.33670701499282,38.2343876482823));
#35456=CARTESIAN_POINT('Ctrl Pts',(4.56510873163454,-0.91687934098516,38.4333205866457));
#35457=CARTESIAN_POINT('Ctrl Pts',(3.23824674115109,3.34583975599457,38.6322535250092));
#35458=CARTESIAN_POINT('Ctrl Pts',(-1.0655501194135,4.53271303067627,38.8311864633726));
#35459=CARTESIAN_POINT('Ctrl Pts',(-4.38978199161124,1.55264300508237,39.030119401736));
#35460=CARTESIAN_POINT('Ctrl Pts',(-3.67846726040206,-2.85477940410947,
39.2290523400994));
#35461=CARTESIAN_POINT('Ctrl Pts',(0.414478853343105,-4.63778895635907,
39.4279852784629));
#35462=CARTESIAN_POINT('Ctrl Pts',(4.12639313890974,-2.15726043097348,39.6269182168263));
#35463=CARTESIAN_POINT('Ctrl Pts',(4.04489462987461,2.30645184786356,39.8258511551898));
#35464=CARTESIAN_POINT('Ctrl Pts',(0.244907848885221,4.64982393177198,40.0247840935532));
#35465=CARTESIAN_POINT('Ctrl Pts',(-3.7802270717933,2.71860821686265,40.2237170319166));
#35466=CARTESIAN_POINT('Ctrl Pts',(-4.33017589256357,-1.71186782838445,
40.4226499702801));
#35467=CARTESIAN_POINT('Ctrl Pts',(-0.899386323495868,-4.56855565825224,
40.6215829086435));
#35468=CARTESIAN_POINT('Ctrl Pts',(3.35823604979678,-3.22546532698901,40.820515847007));
#35469=CARTESIAN_POINT('Ctrl Pts',(4.52857292413312,1.08303189027643,41.0194487853703));
#35470=CARTESIAN_POINT('Ctrl Pts',(1.53585633535487,4.39546725361082,41.2183817237339));
#35471=CARTESIAN_POINT('Ctrl Pts',(-2.86894131305717,3.66794615293081,41.4173146620972));
#35472=CARTESIAN_POINT('Ctrl Pts',(-4.63599876985225,-0.433100961544568,
41.6162476004607));
#35473=CARTESIAN_POINT('Ctrl Pts',(-2.14175477389098,-4.13298614778951,
41.8151805388241));
#35474=CARTESIAN_POINT('Ctrl Pts',(2.32254996080195,-4.03922744535998,42.0141134771876));
#35475=CARTESIAN_POINT('Ctrl Pts',(4.65006593675241,-0.219670421692099,
42.2130895813624));
#35476=CARTESIAN_POINT('Ctrl Pts',(3.35325446895125,2.44428797335999,42.3457547060828));
#35477=CARTESIAN_POINT('Ctrl Pts',(2.28389974637321,3.20599595416551,42.4121088513486));
#35478=CARTESIAN_POINT('Ctrl Pts',(0.611508770536539,3.88132595430304,35.));
#35479=CARTESIAN_POINT('Ctrl Pts',(0.118578222943326,3.92028118933608,35.));
#35480=CARTESIAN_POINT('Ctrl Pts',(-0.330793196286837,3.8649362500333,35.));
#35481=CARTESIAN_POINT('Ctrl Pts',(-1.19936559364089,3.59881466306489,35.));
#35482=CARTESIAN_POINT('Ctrl Pts',(-1.62149749117243,3.37535010249507,35.));
#35483=CARTESIAN_POINT('Ctrl Pts',(-2.36867762403761,2.78818662381047,35.));
#35484=CARTESIAN_POINT('Ctrl Pts',(-2.6932378844351,2.41841696079855,35.));
#35485=CARTESIAN_POINT('Ctrl Pts',(-3.15963245702077,1.58300838024013,35.));
#35486=CARTESIAN_POINT('Ctrl Pts',(-3.27506359737994,1.16827729677819,35.));
#35487=CARTESIAN_POINT('Ctrl Pts',(-3.36041119364516,0.460553542036781,
35.));
#35488=CARTESIAN_POINT('Ctrl Pts',(-3.3545966628611,0.135941322369615,35.));
#35489=CARTESIAN_POINT('Ctrl Pts',(-3.25862262511255,-0.476833139036369,
35.));
#35490=CARTESIAN_POINT('Ctrl Pts',(-3.17389841532412,-0.767201663680286,
35.));
#35491=CARTESIAN_POINT('Ctrl Pts',(-3.05035511918376,-1.03985107319943,
35.));
#35492=CARTESIAN_POINT('Ctrl Pts',(3.9282775211904,0.00261363778016546,
35.9708380071379));
#35493=CARTESIAN_POINT('Ctrl Pts',(3.93118033843727,0.487443495032958,35.9952950051125));
#35494=CARTESIAN_POINT('Ctrl Pts',(3.62292672813806,2.28323870400638,36.086062982542));
#35495=CARTESIAN_POINT('Ctrl Pts',(0.933577472432809,4.55771548976854,36.2431419394252));
#35496=CARTESIAN_POINT('Ctrl Pts',(-3.3305959172111,3.24830235946759,36.4420748777888));
#35497=CARTESIAN_POINT('Ctrl Pts',(-4.53293738673136,-1.04728985028724,
36.6410078161523));
#35498=CARTESIAN_POINT('Ctrl Pts',(-1.56812897439943,-4.38010375485825,
36.8399407545156));
#35499=CARTESIAN_POINT('Ctrl Pts',(2.7129575081135,-3.70599985813041,37.0332163973897));
#35500=CARTESIAN_POINT('Ctrl Pts',(3.93099554165428,-1.19260423393931,37.1601810608092));
#35501=CARTESIAN_POINT('Ctrl Pts',(3.93831984400274,0.00193663700642166,
37.2208347447742));
#35502=CARTESIAN_POINT('Ctrl Pts',(3.07780630188836,-0.968536646922482,
38.));
#35503=CARTESIAN_POINT('Ctrl Pts',(2.99903510824282,-1.34635453962162,38.));
#35504=CARTESIAN_POINT('Ctrl Pts',(2.84886247697082,-1.70893883494449,38.));
#35505=CARTESIAN_POINT('Ctrl Pts',(2.40059258209399,-2.42969373277311,38.));
#35506=CARTESIAN_POINT('Ctrl Pts',(2.07741558654446,-2.77581644702267,38.));
#35507=CARTESIAN_POINT('Ctrl Pts',(1.44890409383044,-3.22190503673451,38.));
#35508=CARTESIAN_POINT('Ctrl Pts',(1.05009098077866,-3.45341296726265,38.));
#35509=CARTESIAN_POINT('Ctrl Pts',(0.0196169452910218,-3.68379679183913,
38.));
#35510=CARTESIAN_POINT('Ctrl Pts',(-0.46849028901934,-3.69578977970723,
38.));
#35511=CARTESIAN_POINT('Ctrl Pts',(-1.28710045430295,-3.56665885634214,
38.));
#35512=CARTESIAN_POINT('Ctrl Pts',(-1.62645567600777,-3.46531472498767,
38.));
#35513=CARTESIAN_POINT('Ctrl Pts',(-2.1711767312706,-3.2135327704138,38.));
#35514=CARTESIAN_POINT('Ctrl Pts',(-2.46327288395651,-3.05058587178992,
38.));
#35515=CARTESIAN_POINT('Ctrl Pts',(-2.77271538323007,-2.7876149603501,38.));
#35516=CARTESIAN_POINT('Ctrl Pts',(-1.4752554566251,-2.865264193787,36.4017031386693));
#35517=CARTESIAN_POINT('Ctrl Pts',(-1.66869427635609,-2.76566720899584,
36.3893221826344));
#35518=CARTESIAN_POINT('Ctrl Pts',(-1.85161275111611,-2.64670560438004,
36.3774197811539));
#35519=CARTESIAN_POINT('Ctrl Pts',(-2.09281079697536,-2.45249159555157,
36.3597902555439));
#35520=CARTESIAN_POINT('Ctrl Pts',(-2.16192269046745,-2.39179020980833,
36.3544830894472));
#35521=CARTESIAN_POINT('Ctrl Pts',(-2.26887596446572,-2.28942515554214,
36.3457533615933));
#35522=CARTESIAN_POINT('Ctrl Pts',(-2.30838825200233,-2.24957969103573,
36.3424043407513));
#35523=CARTESIAN_POINT('Ctrl Pts',(-2.35861129851129,-2.19621614818392,
36.3379699373801));
#35524=CARTESIAN_POINT('Ctrl Pts',(-2.37028355000504,-2.183613633822,36.3369262723467));
#35525=CARTESIAN_POINT('Ctrl Pts',(-2.38916441559391,-2.16289822266887,
36.3352162229861));
#35526=CARTESIAN_POINT('Ctrl Pts',(-2.39643388059001,-2.15484105626593,
36.3345524375081));
#35527=CARTESIAN_POINT('Ctrl Pts',(-2.41037868396717,-2.13922738878082,
36.3332685845929));
#35528=CARTESIAN_POINT('Ctrl Pts',(-2.4170595355309,-2.13167596483264,36.3326487603306));
#35529=CARTESIAN_POINT('Ctrl Pts',(-2.43233722136632,-2.11424330367405,
36.3312203273868));
#35530=CARTESIAN_POINT('Ctrl Pts',(-2.44090943012627,-2.10434081159747,
36.330410705713));
#35531=CARTESIAN_POINT('Ctrl Pts',(-2.46366055643201,-2.077732978578,36.3282398591823));
#35532=CARTESIAN_POINT('Ctrl Pts',(-2.47772967263198,-2.06093505444706,
36.3268741521003));
#35533=CARTESIAN_POINT('Ctrl Pts',(-2.59564432521869,-1.91719733185216,
36.3152262642827));
#35534=CARTESIAN_POINT('Ctrl Pts',(-2.68981555077983,-1.78266448109943,
36.3045561258471));
#35535=CARTESIAN_POINT('Ctrl Pts',(-2.90296655650853,-1.42255880187577,
36.2766451192449));
#35536=CARTESIAN_POINT('Ctrl Pts',(-3.00619697526368,-1.1889757742665,36.2590762793693));
#35537=CARTESIAN_POINT('Ctrl Pts',(-3.09723001100283,-0.892406918471076,
36.2387879909886));
#35538=CARTESIAN_POINT('Ctrl Pts',(-3.11220098758202,-0.838707191176308,
36.2351947135659));
#35539=CARTESIAN_POINT('Ctrl Pts',(-3.12860596231211,-0.77335485671857,
36.2309399339579));
#35540=CARTESIAN_POINT('Ctrl Pts',(-3.1313783140909,-0.762051747337994,
36.23020828139));
#35541=CARTESIAN_POINT('Ctrl Pts',(-3.13560336091536,-0.744413435422304,
36.2290734147302));
#35542=CARTESIAN_POINT('Ctrl Pts',(-3.13709819101134,-0.738088572967554,
36.2286678385843));
#35543=CARTESIAN_POINT('Ctrl Pts',(-3.13984177468579,-0.72632112201274,
36.2279158659925));
#35544=CARTESIAN_POINT('Ctrl Pts',(-3.14109550405649,-0.720879863391161,
36.2275691944005));
#35545=CARTESIAN_POINT('Ctrl Pts',(-3.14390848360291,-0.708524692862517,
36.2267843606805));
#35546=CARTESIAN_POINT('Ctrl Pts',(-3.14545906890058,-0.7016088951856,36.2263467005048));
#35547=CARTESIAN_POINT('Ctrl Pts',(-3.15000053601545,-0.681035719783496,
36.2250494938298));
#35548=CARTESIAN_POINT('Ctrl Pts',(-3.15292541978737,-0.667363725563551,
36.2241936408038));
#35549=CARTESIAN_POINT('Ctrl Pts',(-3.17473630572985,-0.562066480390239,
36.217646818863));
#35550=CARTESIAN_POINT('Ctrl Pts',(-3.18971552183379,-0.469667736758124,
36.2121612808798));
#35551=CARTESIAN_POINT('Ctrl Pts',(-3.22881685393737,-0.137475661207952,
36.1929448764684));
#35552=CARTESIAN_POINT('Ctrl Pts',(-3.23006391976129,0.104198470726065,
36.1798418610527));
#35553=CARTESIAN_POINT('Ctrl Pts',(-3.19454133368619,0.435317819656115,
36.160884215462));
#35554=CARTESIAN_POINT('Ctrl Pts',(-3.18080107331359,0.526401492349101,
36.1555698766831));
#35555=CARTESIAN_POINT('Ctrl Pts',(-3.15243249578763,0.671893889730702,
36.1468294285881));
#35556=CARTESIAN_POINT('Ctrl Pts',(-3.14024503129078,0.726727324839323,
36.1434770969363));
#35557=CARTESIAN_POINT('Ctrl Pts',(-3.12246623469435,0.797883107871334,
36.1390389195492));
#35558=CARTESIAN_POINT('Ctrl Pts',(-3.11816761874797,0.814520425915876,
36.1379948815497));
#35559=CARTESIAN_POINT('Ctrl Pts',(-3.11093724354449,0.841608473586556,
36.1362843746005));
#35560=CARTESIAN_POINT('Ctrl Pts',(-3.10808534167546,0.852080313344894,
36.1356205071843));
#35561=CARTESIAN_POINT('Ctrl Pts',(-3.10248225175357,0.872251734680528,
36.1343366035991));
#35562=CARTESIAN_POINT('Ctrl Pts',(-3.09973833263651,0.881953216784308,
36.1337168111851));
#35563=CARTESIAN_POINT('Ctrl Pts',(-3.09332614644484,0.904224736958464,
36.1322886061585));
#35564=CARTESIAN_POINT('Ctrl Pts',(-3.08962672060242,0.916785548758172,
36.1314791816102));
#35565=CARTESIAN_POINT('Ctrl Pts',(-3.07953558225134,0.950293529925363,
36.129309207357));
#35566=CARTESIAN_POINT('Ctrl Pts',(-3.07300680849741,0.971198389648268,
36.1279441810858));
#35567=CARTESIAN_POINT('Ctrl Pts',(-3.0159472071808,1.14756308465134,36.1163308383265));
#35568=CARTESIAN_POINT('Ctrl Pts',(-2.95387687150754,1.29901325345948,36.105697220258));
#35569=CARTESIAN_POINT('Ctrl Pts',(-2.76697646274527,1.67157634412449,36.0778999850928));
#35570=CARTESIAN_POINT('Ctrl Pts',(-2.62704589908076,1.8838659841783,36.0604107198992));
#35571=CARTESIAN_POINT('Ctrl Pts',(-2.4268025361608,2.12132573757848,36.0400797143045));
#35572=CARTESIAN_POINT('Ctrl Pts',(-2.38874354333528,2.16409303804695,36.0363872694324));
#35573=CARTESIAN_POINT('Ctrl Pts',(-2.34153542950344,2.2143773270336,36.0320314379602));
#35574=CARTESIAN_POINT('Ctrl Pts',(-2.33346121713322,2.22288413378063,36.0312940349814));
#35575=CARTESIAN_POINT('Ctrl Pts',(-2.32082720425748,2.23605034476201,36.0301522142088));
#35576=CARTESIAN_POINT('Ctrl Pts',(-2.31629950050604,2.24074020851906,36.029745388234));
#35577=CARTESIAN_POINT('Ctrl Pts',(-2.30786846486906,2.24942034050592,36.0289922854517));
#35578=CARTESIAN_POINT('Ctrl Pts',(-2.30396903297706,2.2534141685973,36.0286457260504));
#35579=CARTESIAN_POINT('Ctrl Pts',(-2.29511360627042,2.26243694868658,36.0278626538892));
#35580=CARTESIAN_POINT('Ctrl Pts',(-2.290151462035,2.26745974510023,36.0274266337121));
#35581=CARTESIAN_POINT('Ctrl Pts',(-2.27540346167664,2.28229020923059,36.0261387796157));
#35582=CARTESIAN_POINT('Ctrl Pts',(-2.26557067601711,2.29205127353722,36.0252905607156));
#35583=CARTESIAN_POINT('Ctrl Pts',(-2.19153366999279,2.3646062912491,36.0189783980574));
#35584=CARTESIAN_POINT('Ctrl Pts',(-2.12478637581597,2.42476159288578,36.0137036131672));
#35585=CARTESIAN_POINT('Ctrl Pts',(-1.86643674046048,2.63872350758135,35.9943970810265));
#35586=CARTESIAN_POINT('Ctrl Pts',(-1.65997040785983,2.77325803802885,35.981053019721));
#35587=CARTESIAN_POINT('Ctrl Pts',(-1.35827624099663,2.92396860341079,35.961850542876));
#35588=CARTESIAN_POINT('Ctrl Pts',(-1.27463637834816,2.96138598143209,35.9565630524638));
#35589=CARTESIAN_POINT('Ctrl Pts',(-1.1375192048237,3.01584123027732,35.9478627399254));
#35590=CARTESIAN_POINT('Ctrl Pts',(-1.08499093539938,3.03513465362525,35.944522811462));
#35591=CARTESIAN_POINT('Ctrl Pts',(-1.0157326370007,3.05854528327568,35.9400987738295));
#35592=CARTESIAN_POINT('Ctrl Pts',(-0.999432527825012,3.06391035187438,
35.9390561348554));
#35593=CARTESIAN_POINT('Ctrl Pts',(-0.972759502201917,3.07245409982136,
35.9373473443108));
#35594=CARTESIAN_POINT('Ctrl Pts',(-0.962411873305188,3.07571107651609,
35.9366837842103));
#35595=CARTESIAN_POINT('Ctrl Pts',(-0.942414204529635,3.08189466328807,
35.9354000702273));
#35596=CARTESIAN_POINT('Ctrl Pts',(-0.932766472689344,3.08482835053112,
35.9347801579221));
#35597=CARTESIAN_POINT('Ctrl Pts',(-0.910548242818551,3.09147072288122,
35.9333510959763));
#35598=CARTESIAN_POINT('Ctrl Pts',(-0.897968636476481,3.09514808251229,
35.9325409304278));
#35599=CARTESIAN_POINT('Ctrl Pts',(-0.864270272341653,3.10477629925755,
35.9303676766413));
#35600=CARTESIAN_POINT('Ctrl Pts',(-0.84311287625281,3.11058830633781,35.9290000905431));
#35601=CARTESIAN_POINT('Ctrl Pts',(-0.661863218807286,3.15839317942911,
35.917255867631));
#35602=CARTESIAN_POINT('Ctrl Pts',(-0.498840065700016,3.18820543149673,
35.9064838119598));
#35603=CARTESIAN_POINT('Ctrl Pts',(-0.0775209154443138,3.23214251743292,
35.8782184628344));
#35604=CARTESIAN_POINT('Ctrl Pts',(0.181502930681532,3.22797267735349,35.8603879234517));
#35605=CARTESIAN_POINT('Ctrl Pts',(0.487863319199088,3.18601893455163,35.8402195684928));
#35606=CARTESIAN_POINT('Ctrl Pts',(0.538307763061424,3.17788494441735,35.8369327137392));
#35607=CARTESIAN_POINT('Ctrl Pts',(0.599688383849988,3.16648384856296,35.8329920686422));
#35608=CARTESIAN_POINT('Ctrl Pts',(0.610825264923671,3.1643543773893,35.8322794622434));
#35609=CARTESIAN_POINT('Ctrl Pts',(0.628263365765897,3.16092456329657,35.8311676523732));
#35610=CARTESIAN_POINT('Ctrl Pts',(0.634572195913244,3.15966407732031,35.8307662369272));
#35611=CARTESIAN_POINT('Ctrl Pts',(0.646357797563831,3.15727262567872,35.8300179358789));
#35612=CARTESIAN_POINT('Ctrl Pts',(0.651835339067373,3.15614630945402,35.8296708001458));
#35613=CARTESIAN_POINT('Ctrl Pts',(0.664341425809498,3.15354080655823,35.8288796893868));
#35614=CARTESIAN_POINT('Ctrl Pts',(0.671367963211146,3.15205238043466,35.8284362492664));
#35615=CARTESIAN_POINT('Ctrl Pts',(0.692987271204733,3.14739720691011,35.8270749245637));
#35616=CARTESIAN_POINT('Ctrl Pts',(0.707563300445875,3.1441524663894,35.8261613932797));
#35617=CARTESIAN_POINT('Ctrl Pts',(0.850396354165353,3.11131309319946,35.8172470247137));
#35618=CARTESIAN_POINT('Ctrl Pts',(0.976765664063272,3.07398449267316,35.8096553219812));
#35619=CARTESIAN_POINT('Ctrl Pts',(1.28116377243312,2.96339000666203,35.7913234671513));
#35620=CARTESIAN_POINT('Ctrl Pts',(1.45558247647445,2.88172568056682,35.780760304734));
#35621=CARTESIAN_POINT('Ctrl Pts',(1.70654800596999,2.73559036088559,35.7642735856097));
#35622=CARTESIAN_POINT('Ctrl Pts',(1.78910043840985,2.68232698899493,35.7586216402397));
#35623=CARTESIAN_POINT('Ctrl Pts',(1.91698293481149,2.59128356765466,35.7493783783071));
#35624=CARTESIAN_POINT('Ctrl Pts',(1.9639329974732,2.55588353055802,35.745872467841));
#35625=CARTESIAN_POINT('Ctrl Pts',(2.02353954300244,2.508328195338,35.7412594877645));
#35626=CARTESIAN_POINT('Ctrl Pts',(2.03710357511151,2.49732489340492,35.7401985238074));
#35627=CARTESIAN_POINT('Ctrl Pts',(2.05899814435663,2.47926669655605,35.7384672422277));
#35628=CARTESIAN_POINT('Ctrl Pts',(2.06738357303326,2.47227867936313,35.7377996490559));
#35629=CARTESIAN_POINT('Ctrl Pts',(2.0834294887869,2.45876805592077,35.7365133556708));
#35630=CARTESIAN_POINT('Ctrl Pts',(2.09109526081211,2.45225190266198,35.7358949252326));
#35631=CARTESIAN_POINT('Ctrl Pts',(2.10856282331383,2.43726245061999,35.7344766745273));
#35632=CARTESIAN_POINT('Ctrl Pts',(2.11834423121709,2.42876576541529,35.7336758885155));
#35633=CARTESIAN_POINT('Ctrl Pts',(2.14416746548818,2.40605957695487,35.7315440229543));
#35634=CARTESIAN_POINT('Ctrl Pts',(2.16011903659429,2.39174884129328,35.7302087106815));
#35635=CARTESIAN_POINT('Ctrl Pts',(2.28178596952608,2.28038701143607,35.7198793175012));
#35636=CARTESIAN_POINT('Ctrl Pts',(2.38104065298987,2.17654485412815,35.7105913832565));
#35637=CARTESIAN_POINT('Ctrl Pts',(2.60610116272965,1.9072020843764,35.6873192778303));
#35638=CARTESIAN_POINT('Ctrl Pts',(2.72346917200883,1.73547943336091,35.6731209344519));
#35639=CARTESIAN_POINT('Ctrl Pts',(2.86327716762166,1.48140730809603,35.6536685706928));
#35640=CARTESIAN_POINT('Ctrl Pts',(2.90026300488421,1.40762216183968,35.6481915085174));
#35641=CARTESIAN_POINT('Ctrl Pts',(2.95217899339544,1.29329433477463,35.6400426875703));
#35642=CARTESIAN_POINT('Ctrl Pts',(2.96919330260592,1.25373944989675,35.6372828773444));
#35643=CARTESIAN_POINT('Ctrl Pts',(2.9894558456152,1.20390474923328,35.6338900495056));
#35644=CARTESIAN_POINT('Ctrl Pts',(2.99345118547411,1.19393588856406,35.6332155142094));
#35645=CARTESIAN_POINT('Ctrl Pts',(2.99971151516166,1.17808662315959,35.6321498891079));
#35646=CARTESIAN_POINT('Ctrl Pts',(3.00200917756625,1.17221933326814,35.6317568749454));
#35647=CARTESIAN_POINT('Ctrl Pts',(3.00632254169706,1.16110890536614,35.6310154895963));
#35648=CARTESIAN_POINT('Ctrl Pts',(3.00834171820475,1.15586730284646,35.6306669200337));
#35649=CARTESIAN_POINT('Ctrl Pts',(3.01294585228916,1.14382158984963,35.6298685788811));
#35650=CARTESIAN_POINT('Ctrl Pts',(3.01552146961116,1.13701398715773,35.629419370794));
#35651=CARTESIAN_POINT('Ctrl Pts',(3.02233856552016,1.11880964888251,35.6282232474624));
#35652=CARTESIAN_POINT('Ctrl Pts',(3.02653868850251,1.10739740513477,35.6274787377006));
#35653=CARTESIAN_POINT('Ctrl Pts',(3.0568196732153,1.0236610669434,35.6220530591413));
#35654=CARTESIAN_POINT('Ctrl Pts',(3.08037192600609,0.95044167935542,35.6175107525742));
#35655=CARTESIAN_POINT('Ctrl Pts',(3.11097997869764,0.842135496686508,35.6109890728551));
#35656=CARTESIAN_POINT('Ctrl Pts',(3.12010599606352,0.807667834496542,35.6089422944302));
#35657=CARTESIAN_POINT('Ctrl Pts',(3.19099536871426,0.520768915049164,35.5920907939819));
#35658=CARTESIAN_POINT('Ctrl Pts',(3.22258956834844,0.26187146746877,35.5779830578411));
#35659=CARTESIAN_POINT('Ctrl Pts',(3.22277045874783,-0.0322773699741125,
35.5610272103996));
#35660=CARTESIAN_POINT('Ctrl Pts',(3.22224523984713,-0.066533945178146,
35.5590399266099));
#35661=CARTESIAN_POINT('Ctrl Pts',(3.21890748730524,-0.173222058847471,
35.5528027301262));
#35662=CARTESIAN_POINT('Ctrl Pts',(3.21419767276895,-0.245567538508346,
35.5485036776561));
#35663=CARTESIAN_POINT('Ctrl Pts',(3.20514311002084,-0.33697288876932,35.5429577596319));
#35664=CARTESIAN_POINT('Ctrl Pts',(3.20305899040129,-0.356238911551028,
35.541782396898));
#35665=CARTESIAN_POINT('Ctrl Pts',(3.19946716450695,-0.386857263082903,
35.5399037846077));
#35666=CARTESIAN_POINT('Ctrl Pts',(3.1980724597936,-0.398222570088934,35.5392041122974));
#35667=CARTESIAN_POINT('Ctrl Pts',(3.19535127629391,-0.419460375111782,
35.537892182604));
#35668=CARTESIAN_POINT('Ctrl Pts',(3.19403953329945,-0.429334649629104,
35.5372803993823));
#35669=CARTESIAN_POINT('Ctrl Pts',(3.19101107114512,-0.451349357235508,
35.5359123039807));
#35670=CARTESIAN_POINT('Ctrl Pts',(3.18927080993015,-0.463486345758742,
35.5351552527041));
#35671=CARTESIAN_POINT('Ctrl Pts',(3.18396657084568,-0.499034276468238,
35.5329295583531));
#35672=CARTESIAN_POINT('Ctrl Pts',(3.18021382781233,-0.52241582519382,35.5314549444777));
#35673=CARTESIAN_POINT('Ctrl Pts',(3.14448045485697,-0.730378754707215,
35.5182414144364));
#35674=CARTESIAN_POINT('Ctrl Pts',(3.09672586591152,-0.911854036969413,
35.505990195684));
#35675=CARTESIAN_POINT('Ctrl Pts',(2.9656460481618,-1.27727914256669,35.4799597309547));
#35676=CARTESIAN_POINT('Ctrl Pts',(2.88025696302375,-1.45966344587103,35.466189726902));
#35677=CARTESIAN_POINT('Ctrl Pts',(2.73622269328183,-1.70474207114958,35.4473403881831));
#35678=CARTESIAN_POINT('Ctrl Pts',(2.69123067814493,-1.77491978094744,35.4419040066358));
#35679=CARTESIAN_POINT('Ctrl Pts',(2.63578119894601,-1.85444337392499,35.4357656432674));
#35680=CARTESIAN_POINT('Ctrl Pts',(2.62792686323624,-1.86555706765961,35.4349083201578));
#35681=CARTESIAN_POINT('Ctrl Pts',(2.61592162305662,-1.88231791459035,35.4336165957597));
#35682=CARTESIAN_POINT('Ctrl Pts',(2.6118224261631,-1.88800166471346,35.4331787764034));
#35683=CARTESIAN_POINT('Ctrl Pts',(2.6044269530751,-1.89818569295259,35.4323947565128));
#35684=CARTESIAN_POINT('Ctrl Pts',(2.60113751873638,-1.90269080224331,35.4320480952229));
#35685=CARTESIAN_POINT('Ctrl Pts',(2.59395485720042,-1.91247451749451,35.4312956204062));
#35686=CARTESIAN_POINT('Ctrl Pts',(2.5900572199996,-1.91774976996398,35.4308901207858));
#35687=CARTESIAN_POINT('Ctrl Pts',(2.579034956004,-1.93257294270851,35.4297512096261));
#35688=CARTESIAN_POINT('Ctrl Pts',(2.57187336579427,-1.94209342818767,35.4290203320154));
#35689=CARTESIAN_POINT('Ctrl Pts',(2.52804589648987,-1.99968924852045,35.4246010107285));
#35690=CARTESIAN_POINT('Ctrl Pts',(2.49008323391232,-2.04676811675291,35.4209981831955));
#35691=CARTESIAN_POINT('Ctrl Pts',(2.28489354975244,-2.28706488110814,35.40249454867));
#35692=CARTESIAN_POINT('Ctrl Pts',(2.09643850884567,-2.46097052873984,35.3886395806164));
#35693=CARTESIAN_POINT('Ctrl Pts',(1.76143196867848,-2.70341046135735,35.3652458027176));
#35694=CARTESIAN_POINT('Ctrl Pts',(1.62684207387483,-2.78647554838319,35.356126270503));
#35695=CARTESIAN_POINT('Ctrl Pts',(1.467387265963,-2.86938439405468,35.3453154817556));
#35696=CARTESIAN_POINT('Ctrl Pts',(1.44795700712991,-2.87923820809416,35.3439983244115));
#35697=CARTESIAN_POINT('Ctrl Pts',(1.41672087715647,-2.89468307490204,35.3418804623409));
#35698=CARTESIAN_POINT('Ctrl Pts',(1.40497811468858,-2.90040077183462,35.3410841959532));
#35699=CARTESIAN_POINT('Ctrl Pts',(1.38411443619748,-2.91040312218429,35.339669150958));
#35700=CARTESIAN_POINT('Ctrl Pts',(1.37500751912376,-2.91471669717657,35.3390513897142));
#35701=CARTESIAN_POINT('Ctrl Pts',(1.3560369876221,-2.92359357021239,35.3377642617047));
#35702=CARTESIAN_POINT('Ctrl Pts',(1.34617023405761,-2.92814982060188,35.3370946603137));
#35703=CARTESIAN_POINT('Ctrl Pts',(1.32058308736153,-2.93980874357326,35.3353577093626));
#35704=CARTESIAN_POINT('Ctrl Pts',(1.30482853168874,-2.94683518773189,35.3342877496162));
#35705=CARTESIAN_POINT('Ctrl Pts',(1.23698173352815,-2.9764437312877,35.3296773755474));
#35706=CARTESIAN_POINT('Ctrl Pts',(1.18435676770846,-2.99777241964207,35.3260945593449));
#35707=CARTESIAN_POINT('Ctrl Pts',(1.04366031753545,-3.05051313782734,35.3164915764213));
#35708=CARTESIAN_POINT('Ctrl Pts',(0.954743117662606,-3.07949999194473,
35.3103969897814));
#35709=CARTESIAN_POINT('Ctrl Pts',(0.656845778650454,-3.16247139270354,
35.2899247795844));
#35710=CARTESIAN_POINT('Ctrl Pts',(0.443710345811826,-3.199340739048,35.2751505480742));
#35711=CARTESIAN_POINT('Ctrl Pts',(0.113232386153195,-3.22283315364041,
35.2529448366808));
#35712=CARTESIAN_POINT('Ctrl Pts',(-0.00242276030634944,-3.22482174519131,
35.2453152469946));
#35713=CARTESIAN_POINT('Ctrl Pts',(-0.132683918455096,-3.2200512461733,
35.2370526009332));
#35714=CARTESIAN_POINT('Ctrl Pts',(-0.147417957322412,-3.21941035215556,
35.2361228164553));
#35715=CARTESIAN_POINT('Ctrl Pts',(-0.169284399981222,-3.21830878263779,
35.2347506128558));
#35716=CARTESIAN_POINT('Ctrl Pts',(-0.176420262156259,-3.21792549974631,
35.2343040230992));
#35717=CARTESIAN_POINT('Ctrl Pts',(-0.189134577961852,-3.21720016603975,
35.2335105456669));
#35718=CARTESIAN_POINT('Ctrl Pts',(-0.194713460213433,-3.21686733749034,
35.2331631481637));
#35719=CARTESIAN_POINT('Ctrl Pts',(-0.206736929684483,-3.21611864022215,
35.2324161189759));
#35720=CARTESIAN_POINT('Ctrl Pts',(-0.213181122619191,-3.2156979144143,
35.2320167632884));
#35721=CARTESIAN_POINT('Ctrl Pts',(-0.23104695915257,-3.21447755572762,
35.2309123357424));
#35722=CARTESIAN_POINT('Ctrl Pts',(-0.242465805131233,-3.21363641318313,
35.2302095577113));
#35723=CARTESIAN_POINT('Ctrl Pts',(-0.30647150506476,-3.20857848651103,
35.2262865344371));
#35724=CARTESIAN_POINT('Ctrl Pts',(-0.358956472586155,-3.20313154328421,
35.2231311068008));
#35725=CARTESIAN_POINT('Ctrl Pts',(-0.665949292365562,-3.16363011399075,
35.2049125407654));
#35726=CARTESIAN_POINT('Ctrl Pts',(-0.915807722760667,-3.10054341059219,
35.1909852445635));
#35727=CARTESIAN_POINT('Ctrl Pts',(-1.2646773558253,-2.96654253713258,35.1698817324028));
#35728=CARTESIAN_POINT('Ctrl Pts',(-1.37140074843424,-2.91873648247267,
35.1631909462925));
#35729=CARTESIAN_POINT('Ctrl Pts',(-1.4752555264658,-2.86526415782771,35.1563175586878));
#35730=CARTESIAN_POINT('Origin',(0.,0.,4.68922655072688));
#35731=CARTESIAN_POINT('',(3.22274857165764,-0.00244669484556194,35.3125278845694));
#35732=CARTESIAN_POINT('Ctrl Pts',(3.22274907127793,-0.00244664611808667,
35.3125270209625));
#35733=CARTESIAN_POINT('Ctrl Pts',(3.222822198994,0.0938779826516697,35.3180030298239));
#35734=CARTESIAN_POINT('Ctrl Pts',(3.2185767818221,0.190152796939803,35.3235561489518));
#35735=CARTESIAN_POINT('Ctrl Pts',(3.20588205807585,0.332591966317148,35.3319873302714));
#35736=CARTESIAN_POINT('Ctrl Pts',(3.20072779093437,0.378996656346596,35.3347679097327));
#35737=CARTESIAN_POINT('Ctrl Pts',(3.19245693920111,0.441125918843006,35.3385432245935));
#35738=CARTESIAN_POINT('Ctrl Pts',(3.19022835540884,0.456964343398726,35.3395102459607));
#35739=CARTESIAN_POINT('Ctrl Pts',(3.18626032428469,0.483719859681448,35.3411518760625));
#35740=CARTESIAN_POINT('Ctrl Pts',(3.18458242116393,0.494645888305743,35.3418245401713));
#35741=CARTESIAN_POINT('Ctrl Pts',(3.18138073222578,0.514802606888697,35.343069798848));
#35742=CARTESIAN_POINT('Ctrl Pts',(3.17987289518586,0.524035738267946,35.3436418822315));
#35743=CARTESIAN_POINT('Ctrl Pts',(3.17667380192803,0.543102830753287,35.3448267903223));
#35744=CARTESIAN_POINT('Ctrl Pts',(3.17497703570969,0.552935753749137,35.3454397847159));
#35745=CARTESIAN_POINT('Ctrl Pts',(3.17104917621089,0.575083752271063,35.3468249504617));
#35746=CARTESIAN_POINT('Ctrl Pts',(3.16879196380773,0.587393976037243,35.347597947873));
#35747=CARTESIAN_POINT('Ctrl Pts',(3.16283206722838,0.61886319151895,35.3495820765352));
#35748=CARTESIAN_POINT('Ctrl Pts',(3.15902701529105,0.63800205714112,35.3507964632919));
#35749=CARTESIAN_POINT('Ctrl Pts',(3.13493297705785,0.753688096794359,35.3581845259994));
#35750=CARTESIAN_POINT('Ctrl Pts',(3.11039519341025,0.849287276382102,35.3644936335693));
#35751=CARTESIAN_POINT('Ctrl Pts',(3.06261102411507,1.00533551957057,35.3751383797574));
#35752=CARTESIAN_POINT('Ctrl Pts',(3.0418578526508,1.06648292520211,35.379399773773));
#35753=CARTESIAN_POINT('Ctrl Pts',(2.94398912463826,1.32868619866432,35.3980416007017));
#35754=CARTESIAN_POINT('Ctrl Pts',(2.84867416605034,1.52234281914099,35.4128122584179));
#35755=CARTESIAN_POINT('Ctrl Pts',(2.68796576556024,1.78010743066332,35.4330477547681));
#35756=CARTESIAN_POINT('Ctrl Pts',(2.63809033463233,1.85322009616731,35.4388531537061));
#35757=CARTESIAN_POINT('Ctrl Pts',(2.5738869008461,1.93948110285755,35.4457007292539));
#35758=CARTESIAN_POINT('Ctrl Pts',(2.5623729990046,1.9546675885902,35.4469061530209));
#35759=CARTESIAN_POINT('Ctrl Pts',(2.54587837315102,1.97602726308972,35.4486003580822));
#35760=CARTESIAN_POINT('Ctrl Pts',(2.54100879890514,1.98228522730869,35.449096577208));
#35761=CARTESIAN_POINT('Ctrl Pts',(2.53260068933571,1.99300872320809,35.4499465348641));
#35762=CARTESIAN_POINT('Ctrl Pts',(2.5290733341092,1.99748293987475,35.4503010600482));
#35763=CARTESIAN_POINT('Ctrl Pts',(2.52222693279569,2.00611993793479,35.4509851924609));
#35764=CARTESIAN_POINT('Ctrl Pts',(2.51890943473924,2.01028385221078,35.4513149097283));
#35765=CARTESIAN_POINT('Ctrl Pts',(2.50996017443316,2.02145946404088,35.4521996216935));
#35766=CARTESIAN_POINT('Ctrl Pts',(2.50430930530922,2.02845590286812,35.4527532546306));
#35767=CARTESIAN_POINT('Ctrl Pts',(2.4833899848165,2.05413581198401,35.454784834301));
#35768=CARTESIAN_POINT('Ctrl Pts',(2.46794069348604,2.07267184186707,35.4562502916358));
#35769=CARTESIAN_POINT('Ctrl Pts',(2.32053141693219,2.24554782791318,35.469927795437));
#35770=CARTESIAN_POINT('Ctrl Pts',(2.17445047837928,2.38728703534737,35.4812353044151));
#35771=CARTESIAN_POINT('Ctrl Pts',(1.88435771502452,2.61988086240072,35.5020094141611));
#35772=CARTESIAN_POINT('Ctrl Pts',(1.74465664835936,2.71491207884529,35.5114319292465));
#35773=CARTESIAN_POINT('Ctrl Pts',(1.5464281871252,2.82811377439754,35.5246682146053));
#35774=CARTESIAN_POINT('Ctrl Pts',(1.4938808924124,2.85621898990891,35.5281632300493));
#35775=CARTESIAN_POINT('Ctrl Pts',(1.41606868102879,2.89510246998893,35.5333379420563));
#35776=CARTESIAN_POINT('Ctrl Pts',(1.3913956644315,2.90704091091488,35.5349786056314));
#35777=CARTESIAN_POINT('Ctrl Pts',(1.34675667191248,2.92794174274711,35.5379484416452));
#35778=CARTESIAN_POINT('Ctrl Pts',(1.32684582374589,2.93701830193329,35.5392736405939));
#35779=CARTESIAN_POINT('Ctrl Pts',(1.29603469935726,2.95068660944577,35.541325790494));
#35780=CARTESIAN_POINT('Ctrl Pts',(1.28519874229726,2.9554224056854,35.5420477859514));
#35781=CARTESIAN_POINT('Ctrl Pts',(1.26608673208441,2.96365022108519,35.5433217974865));
#35782=CARTESIAN_POINT('Ctrl Pts',(1.25782164012358,2.96716749866542,35.5438729422159));
#35783=CARTESIAN_POINT('Ctrl Pts',(1.23917063255296,2.97501265594226,35.5451171384687));
#35784=CARTESIAN_POINT('Ctrl Pts',(1.22877657943962,2.97932077364512,35.5458108548017));
#35785=CARTESIAN_POINT('Ctrl Pts',(1.20077530730874,2.9907552592962,35.5476807175804));
#35786=CARTESIAN_POINT('Ctrl Pts',(1.18312750074961,2.99778045421981,35.5488602712433));
#35787=CARTESIAN_POINT('Ctrl Pts',(1.10360230784894,3.02862604087624,35.5541811551656));
#35788=CARTESIAN_POINT('Ctrl Pts',(1.0410645080087,3.05068801941584,35.5583808882861));
#35789=CARTESIAN_POINT('Ctrl Pts',(0.670324953753376,3.16874962926328,35.5833851699237));
#35790=CARTESIAN_POINT('Ctrl Pts',(0.349804969398493,3.21991791190272,35.6056886694998));
#35791=CARTESIAN_POINT('Ctrl Pts',(-0.0350210707554559,3.22315930273634,
35.6312791652481));
#35792=CARTESIAN_POINT('Ctrl Pts',(-0.0971925808733141,3.22188406580124,
35.6353675708624));
#35793=CARTESIAN_POINT('Ctrl Pts',(-0.182893561452371,3.21764291224097,
35.6409071917649));
#35794=CARTESIAN_POINT('Ctrl Pts',(-0.206482432798357,3.21621532886052,
35.6424218546974));
#35795=CARTESIAN_POINT('Ctrl Pts',(-0.247231118304599,3.21329906704435,
35.6450184917643));
#35796=CARTESIAN_POINT('Ctrl Pts',(-0.264398353381229,3.21193207610899,
35.646106333131));
#35797=CARTESIAN_POINT('Ctrl Pts',(-0.289135386438601,3.20976264022414,
35.6476642406725));
#35798=CARTESIAN_POINT('Ctrl Pts',(-0.296714242463301,3.20907091529585,
35.6481402449312));
#35799=CARTESIAN_POINT('Ctrl Pts',(-0.309910016238329,3.20781938479212,
35.6489666766877));
#35800=CARTESIAN_POINT('Ctrl Pts',(-0.31552801204594,3.2072716597146,35.6493177779765));
#35801=CARTESIAN_POINT('Ctrl Pts',(-0.327307768498945,3.20609194379902,
35.6500523711005));
#35802=CARTESIAN_POINT('Ctrl Pts',(-0.333469149909224,3.20545694948554,
35.6504356918027));
#35803=CARTESIAN_POINT('Ctrl Pts',(-0.349836035200082,3.20372247086048,
35.6514516121746));
#35804=CARTESIAN_POINT('Ctrl Pts',(-0.360038282121318,3.20259197586956,
35.6520824847972));
#35805=CARTESIAN_POINT('Ctrl Pts',(-0.40367289845304,3.19754574518788,35.6547711014066));
#35806=CARTESIAN_POINT('Ctrl Pts',(-0.437049586291402,3.19315493961492,
35.6568035218393));
#35807=CARTESIAN_POINT('Ctrl Pts',(-0.476615547774752,3.18731787825588,
35.6591906079939));
#35808=CARTESIAN_POINT('Ctrl Pts',(-0.482875551191465,3.1863755021517,35.6595676223802));
#35809=CARTESIAN_POINT('Ctrl Pts',(-0.78807014476277,3.13951168803674,35.6779176620613));
#35810=CARTESIAN_POINT('Ctrl Pts',(-1.07909311969837,3.05175323564138,35.6941078273691));
#35811=CARTESIAN_POINT('Ctrl Pts',(-1.43660826328232,2.88628354462794,35.7165410559189));
#35812=CARTESIAN_POINT('Ctrl Pts',(-1.51789998880267,2.84437228964257,35.7218192810321));
#35813=CARTESIAN_POINT('Ctrl Pts',(-1.64582570326363,2.77137102702872,35.7305055138283));
#35814=CARTESIAN_POINT('Ctrl Pts',(-1.69362443773071,2.74242143171488,35.7338409247734));
#35815=CARTESIAN_POINT('Ctrl Pts',(-1.7550761634918,2.70298340343429,35.7382595874149));
#35816=CARTESIAN_POINT('Ctrl Pts',(-1.76943349387717,2.69360663645655,35.7393014896748));
#35817=CARTESIAN_POINT('Ctrl Pts',(-1.79274581969509,2.67811455287119,35.7410092249677));
#35818=CARTESIAN_POINT('Ctrl Pts',(-1.80174611087036,2.67206775358597,35.7416724710425));
#35819=CARTESIAN_POINT('Ctrl Pts',(-1.81905491081398,2.66031171451251,35.7429556837871));
#35820=CARTESIAN_POINT('Ctrl Pts',(-1.82736749378812,2.65460867660189,35.7435754096296));
#35821=CARTESIAN_POINT('Ctrl Pts',(-1.8464241598826,2.64140249025563,35.745004193069));
#35822=CARTESIAN_POINT('Ctrl Pts',(-1.85714945377346,2.63387266053652,35.7458142669076));
#35823=CARTESIAN_POINT('Ctrl Pts',(-1.88571089358673,2.6135595504263,35.7479876068367));
#35824=CARTESIAN_POINT('Ctrl Pts',(-1.90346265497794,2.60065933571649,35.7493553731951));
#35825=CARTESIAN_POINT('Ctrl Pts',(-2.05259145839286,2.48994252587534,35.7609923150584));
#35826=CARTESIAN_POINT('Ctrl Pts',(-2.17644666712245,2.38243797731905,35.7716483608506));
#35827=CARTESIAN_POINT('Ctrl Pts',(-2.47009394478667,2.0854759631843,35.7995028679659));
#35828=CARTESIAN_POINT('Ctrl Pts',(-2.62663991601537,1.8844978151653,35.8170272932151));
#35829=CARTESIAN_POINT('Ctrl Pts',(-2.78717237984905,1.61894177903155,35.8373288032252));
#35830=CARTESIAN_POINT('Ctrl Pts',(-2.81509616944046,1.56988433892823,35.8409682944937));
#35831=CARTESIAN_POINT('Ctrl Pts',(-2.84722706337797,1.50981852463014,35.8452700206613));
#35832=CARTESIAN_POINT('Ctrl Pts',(-2.8526792567236,1.49949157912259,35.8460041995074));
#35833=CARTESIAN_POINT('Ctrl Pts',(-2.86108165915521,1.48336496995739,35.8471420350367));
#35834=CARTESIAN_POINT('Ctrl Pts',(-2.86407057471238,1.47758574685005,35.8475480744458));
#35835=CARTESIAN_POINT('Ctrl Pts',(-2.86959073405829,1.46683254934182,35.8483003279048));
#35836=CARTESIAN_POINT('Ctrl Pts',(-2.87212653543665,1.46186109940702,35.8486468205337));
#35837=CARTESIAN_POINT('Ctrl Pts',(-2.87784626086216,1.45057521985763,35.8494305058163));
#35838=CARTESIAN_POINT('Ctrl Pts',(-2.88102231595407,1.44425689780227,35.8498672014981));
#35839=CARTESIAN_POINT('Ctrl Pts',(-2.89038546486611,1.42547641484685,35.8511593211402));
#35840=CARTESIAN_POINT('Ctrl Pts',(-2.89651277506788,1.41298439653568,35.8520110931471));
#35841=CARTESIAN_POINT('Ctrl Pts',(-2.94236488448253,1.31795195014025,35.8584356891103));
#35842=CARTESIAN_POINT('Ctrl Pts',(-2.97863920195295,1.23378293082401,35.8638116284189));
#35843=CARTESIAN_POINT('Ctrl Pts',(-3.09796907748042,0.920820293972021,
35.8830722180209));
#35844=CARTESIAN_POINT('Ctrl Pts',(-3.15863409748303,0.684372923629414,
35.896298481329));
#35845=CARTESIAN_POINT('Ctrl Pts',(-3.20474754755038,0.352348715279247,
35.9153828810517));
#35846=CARTESIAN_POINT('Ctrl Pts',(-3.21348774603249,0.260865942913228,
35.9206853786294));
#35847=CARTESIAN_POINT('Ctrl Pts',(-3.22125103730935,0.113149652394659,
35.9294079034964));
#35848=CARTESIAN_POINT('Ctrl Pts',(-3.22273185991701,0.0570952960618219,
35.9327545369201));
#35849=CARTESIAN_POINT('Ctrl Pts',(-3.22275533909513,-0.0161359277741507,
35.9371859942254));
#35850=CARTESIAN_POINT('Ctrl Pts',(-3.22262364041845,-0.0333046288324061,
35.9382291637872));
#35851=CARTESIAN_POINT('Ctrl Pts',(-3.22218487970022,-0.0613174874208513,
35.9399384538424));
#35852=CARTESIAN_POINT('Ctrl Pts',(-3.22196023686762,-0.0721627377965504,
35.9406019782694));
#35853=CARTESIAN_POINT('Ctrl Pts',(-3.22142124196038,-0.0930824086395146,
35.9418853624112));
#35854=CARTESIAN_POINT('Ctrl Pts',(-3.2211143726453,-0.10315690769907,35.9425049793255));
#35855=CARTESIAN_POINT('Ctrl Pts',(-3.22030020351147,-0.126315525354007,
35.9439329850104));
#35856=CARTESIAN_POINT('Ctrl Pts',(-3.21976041510896,-0.139398256247839,
35.9447423864189));
#35857=CARTESIAN_POINT('Ctrl Pts',(-3.21810443471131,-0.174359777866476,
35.9469127498439));
#35858=CARTESIAN_POINT('Ctrl Pts',(-3.21684487112074,-0.196230786862113,
35.948278192795));
#35859=CARTESIAN_POINT('Ctrl Pts',(-3.20426121056356,-0.381757946721685,
35.9599284392866));
#35860=CARTESIAN_POINT('Ctrl Pts',(-3.18068132286312,-0.544316657537262,
35.9706014164879));
#35861=CARTESIAN_POINT('Ctrl Pts',(-3.0892667155855,-0.952469482132061,
35.998499587124));
#35862=CARTESIAN_POINT('Ctrl Pts',(-3.00453278854938,-1.19312402986472,
36.0160512963132));
#35863=CARTESIAN_POINT('Ctrl Pts',(-2.86773749741407,-1.47150484730143,
36.0363383813135));
#35864=CARTESIAN_POINT('Ctrl Pts',(-2.84177029808648,-1.52104810623624,
36.0399440790494));
#35865=CARTESIAN_POINT('Ctrl Pts',(-2.80885164644733,-1.58006507235858,
36.0442113504063));
#35866=CARTESIAN_POINT('Ctrl Pts',(-2.8031230808684,-1.59020571245238,36.0449435571804));
#35867=CARTESIAN_POINT('Ctrl Pts',(-2.79411210041919,-1.60595684151635,
36.0460790076063));
#35868=CARTESIAN_POINT('Ctrl Pts',(-2.7908675420878,-1.61158871019074,36.0464846181944));
#35869=CARTESIAN_POINT('Ctrl Pts',(-2.78480502505577,-1.62203874467475,
36.0472364846307));
#35870=CARTESIAN_POINT('Ctrl Pts',(-2.78199161484652,-1.62685935852861,
36.0475830165017));
#35871=CARTESIAN_POINT('Ctrl Pts',(-2.77558059952186,-1.63777899505023,
36.0483673095912));
#35872=CARTESIAN_POINT('Ctrl Pts',(-2.77197541752484,-1.64387347079022,
36.0488045706096));
#35873=CARTESIAN_POINT('Ctrl Pts',(-2.76120457265491,-1.66194514565416,
36.0500999161951));
#35874=CARTESIAN_POINT('Ctrl Pts',(-2.75398105038895,-1.67388791430352,
36.050954321706));
#35875=CARTESIAN_POINT('Ctrl Pts',(-2.69807807434776,-1.76497171935793,
36.0574610713057));
#35876=CARTESIAN_POINT('Ctrl Pts',(-2.64606923707545,-1.84202919295389,
36.0629107944885));
#35877=CARTESIAN_POINT('Ctrl Pts',(-2.44705131726415,-2.11103574983077,
36.0821409989197));
#35878=CARTESIAN_POINT('Ctrl Pts',(-2.28190073615814,-2.28855277342994,
36.0952837718125));
#35879=CARTESIAN_POINT('Ctrl Pts',(-2.02860552848562,-2.50586217024917,
36.1142829562129));
#35880=CARTESIAN_POINT('Ctrl Pts',(-1.95623474136634,-2.56275814472599,
36.119594215877));
#35881=CARTESIAN_POINT('Ctrl Pts',(-1.83595694390226,-2.6492510166241,36.1283298372918));
#35882=CARTESIAN_POINT('Ctrl Pts',(-1.78953488430647,-2.68082695623838,
36.1316805162257));
#35883=CARTESIAN_POINT('Ctrl Pts',(-1.72786376367948,-2.72045941322018,
36.1361165850886));
#35884=CARTESIAN_POINT('Ctrl Pts',(-1.71333981160578,-2.7296298791251,36.1371602105065));
#35885=CARTESIAN_POINT('Ctrl Pts',(-1.68952376613095,-2.74440243281156,
36.1388700598438));
#35886=CARTESIAN_POINT('Ctrl Pts',(-1.68027534400173,-2.75007455050425,
36.1395336844176));
#35887=CARTESIAN_POINT('Ctrl Pts',(-1.66238055990656,-2.7609255721317,36.140817130465));
#35888=CARTESIAN_POINT('Ctrl Pts',(-1.65373818681447,-2.76611083411253,
36.1414367084293));
#35889=CARTESIAN_POINT('Ctrl Pts',(-1.63381552198751,-2.77793731968781,
36.1428644354347));
#35890=CARTESIAN_POINT('Ctrl Pts',(-1.62251886347597,-2.784550491828,36.1436735958224));
#35891=CARTESIAN_POINT('Ctrl Pts',(-1.59222088829513,-2.80204024783262,
36.145842892712));
#35892=CARTESIAN_POINT('Ctrl Pts',(-1.57314875726316,-2.81279218160706,
36.1472075032309));
#35893=CARTESIAN_POINT('Ctrl Pts',(-1.52791931900792,-2.83768642883583,
36.1504420200467));
#35894=CARTESIAN_POINT('Ctrl Pts',(-1.50167885936097,-2.85165942216976,
36.1523172954271));
#35895=CARTESIAN_POINT('Ctrl Pts',(-1.47525533429856,-2.86526425676998,
36.1542047394732));
#35896=CARTESIAN_POINT('',(-0.0206799398372109,-3.22268774565723,34.9999898625471));
#35897=CARTESIAN_POINT('Ctrl Pts',(-0.0206996961560602,-3.22268352232717,
34.9999891441435));
#35898=CARTESIAN_POINT('Ctrl Pts',(0.119331606346545,-3.22358296075917,
35.0094451984274));
#35899=CARTESIAN_POINT('Ctrl Pts',(0.25936552548738,-3.21535540382481,35.0189818957179));
#35900=CARTESIAN_POINT('Ctrl Pts',(0.418350219005723,-3.19554380295184,
35.0296712679666));
#35901=CARTESIAN_POINT('Ctrl Pts',(0.438162186753174,-3.19288756849992,
35.0310006946464));
#35902=CARTESIAN_POINT('Ctrl Pts',(0.538410711821889,-3.17849635255725,
35.0377104753343));
#35903=CARTESIAN_POINT('Ctrl Pts',(0.618415001021133,-3.16390431477802,
35.0430099104089));
#35904=CARTESIAN_POINT('Ctrl Pts',(0.710989412689877,-3.14337310041445,
35.0490132261124));
#35905=CARTESIAN_POINT('Ctrl Pts',(0.724171874476634,-3.14036232060865,
35.0498649965779));
#35906=CARTESIAN_POINT('Ctrl Pts',(0.744137358248051,-3.1356699409744,35.0511499399372));
#35907=CARTESIAN_POINT('Ctrl Pts',(0.750934309816619,-3.13404914626411,
35.0515864797157));
#35908=CARTESIAN_POINT('Ctrl Pts',(0.763144882370624,-3.13109542068199,
35.0523690271339));
#35909=CARTESIAN_POINT('Ctrl Pts',(0.768560335508649,-3.12977054383343,
35.0527154888963));
#35910=CARTESIAN_POINT('Ctrl Pts',(0.780350562240213,-3.12685364745952,
35.0534684685532));
#35911=CARTESIAN_POINT('Ctrl Pts',(0.786723894018734,-3.12525618934163,
35.0538746676402));
#35912=CARTESIAN_POINT('Ctrl Pts',(0.80469689099108,-3.12069284333201,35.0550179272153));
#35913=CARTESIAN_POINT('Ctrl Pts',(0.816285121816515,-3.11768175398948,
35.0557524216429));
#35914=CARTESIAN_POINT('Ctrl Pts',(0.887394488285968,-3.09878101651963,
35.060244858625));
#35915=CARTESIAN_POINT('Ctrl Pts',(0.946471035216613,-3.0812508002563,35.063913850737));
#35916=CARTESIAN_POINT('Ctrl Pts',(1.25864133498492,-2.97879114230051,35.0831396542036));
#35917=CARTESIAN_POINT('Ctrl Pts',(1.50096483369849,-2.86435117756486,35.0975670168958));
#35918=CARTESIAN_POINT('Ctrl Pts',(1.84950045737443,-2.64323899408243,35.120997180681));
#35919=CARTESIAN_POINT('Ctrl Pts',(1.96713019752114,-2.55690344213947,35.1294438775362));
#35920=CARTESIAN_POINT('Ctrl Pts',(2.09496623624399,-2.44901979951021,35.1395081131937));
#35921=CARTESIAN_POINT('Ctrl Pts',(2.11128724137151,-2.43496358479719,35.1408105703398));
#35922=CARTESIAN_POINT('Ctrl Pts',(2.13722039559061,-2.41217229639306,35.1429091243416));
#35923=CARTESIAN_POINT('Ctrl Pts',(2.14692294891978,-2.40354073201732,35.1437009098924));
#35924=CARTESIAN_POINT('Ctrl Pts',(2.16405060814628,-2.38811720508672,35.1451106139376));
#35925=CARTESIAN_POINT('Ctrl Pts',(2.1714966111556,-2.38134862713143,35.1457275392704));
#35926=CARTESIAN_POINT('Ctrl Pts',(2.18577929560792,-2.36824266797561,35.14691885616));
#35927=CARTESIAN_POINT('Ctrl Pts',(2.19262042788094,-2.36191026921959,35.1474930313998));
#35928=CARTESIAN_POINT('Ctrl Pts',(2.21046113508075,-2.34525195816643,35.1489998132359));
#35929=CARTESIAN_POINT('Ctrl Pts',(2.22141574557196,-2.33487842292567,35.1499344685525));
#35930=CARTESIAN_POINT('Ctrl Pts',(2.26262368632985,-2.29530380858307,35.1534867380244));
#35931=CARTESIAN_POINT('Ctrl Pts',(2.29237629209639,-2.2655895888391,35.1561267090831));
#35932=CARTESIAN_POINT('Ctrl Pts',(2.36498724047232,-2.19017740471364,35.1627633713943));
#35933=CARTESIAN_POINT('Ctrl Pts',(2.40710902354072,-2.14379733402282,35.1667898613596));
#35934=CARTESIAN_POINT('Ctrl Pts',(2.52683000432368,-2.00399387390788,35.1787689156205));
#35935=CARTESIAN_POINT('Ctrl Pts',(2.60052735404878,-1.9073841069181,35.1868540777386));
#35936=CARTESIAN_POINT('Ctrl Pts',(2.80829628852151,-1.60052450429051,35.2118120830906));
#35937=CARTESIAN_POINT('Ctrl Pts',(2.92360460029175,-1.37867950457497,35.2289539029287));
#35938=CARTESIAN_POINT('Ctrl Pts',(3.01975798738673,-1.12589116364772,35.2462198111673));
#35939=CARTESIAN_POINT('Ctrl Pts',(3.02711712655888,-1.1059526089785,35.2475666645863));
#35940=CARTESIAN_POINT('Ctrl Pts',(3.03715400392429,-1.07790812734312,35.2494387003354));
#35941=CARTESIAN_POINT('Ctrl Pts',(3.03999741382545,-1.06986265586188,35.2499731902159));
#35942=CARTESIAN_POINT('Ctrl Pts',(3.04453383113319,-1.05686267995059,35.250832584171));
#35943=CARTESIAN_POINT('Ctrl Pts',(3.04624675537791,-1.05191524348307,35.2511586578931));
#35944=CARTESIAN_POINT('Ctrl Pts',(3.0498223232361,-1.04150595757504,35.2518426002686));
#35945=CARTESIAN_POINT('Ctrl Pts',(3.05168236362497,-1.03604324970668,35.2522003070227));
#35946=CARTESIAN_POINT('Ctrl Pts',(3.05618729722679,-1.02269542692598,35.2530714324032));
#35947=CARTESIAN_POINT('Ctrl Pts',(3.05881638239471,-1.01480494401201,35.2535839185662));
#35948=CARTESIAN_POINT('Ctrl Pts',(3.06812182888641,-0.98651245021176,35.2554129612008));
#35949=CARTESIAN_POINT('Ctrl Pts',(3.07462502953678,-0.966053495529832,
35.2567196951894));
#35950=CARTESIAN_POINT('Ctrl Pts',(3.11354420921741,-0.839238949451706,
35.264730398011));
#35951=CARTESIAN_POINT('Ctrl Pts',(3.14064605225898,-0.73131878439612,35.2711631847051));
#35952=CARTESIAN_POINT('Ctrl Pts',(3.20228605224234,-0.418056310754366,
35.2892997880465));
#35953=CARTESIAN_POINT('Ctrl Pts',(3.22259086965953,-0.210506202816104,
35.3006989395904));
#35954=CARTESIAN_POINT('Ctrl Pts',(3.2227490683711,-0.00245047203661506,
35.3125268034609));
#35955=CARTESIAN_POINT('Origin',(0.,0.,35.));
#35956=CARTESIAN_POINT('Origin',(0.,0.,32.));
#35957=CARTESIAN_POINT('Ctrl Pts',(3.9378436511043,0.00226769081060172,
37.4041617293967));
#35958=CARTESIAN_POINT('Ctrl Pts',(3.92969352726255,-1.17026837568043,37.3446443126903));
#35959=CARTESIAN_POINT('Ctrl Pts',(2.75095850512379,-3.66336727924014,37.2188159165294));
#35960=CARTESIAN_POINT('Ctrl Pts',(-1.49285278529501,-4.40632793330521,
37.026676540914));
#35961=CARTESIAN_POINT('Ctrl Pts',(-4.51432818846032,-1.12480055766829,
36.8277436025506));
#35962=CARTESIAN_POINT('Ctrl Pts',(-3.38576122948677,3.19076106622442,36.6288106641873));
#35963=CARTESIAN_POINT('Ctrl Pts',(0.855351370873146,4.57304158308359,36.4298777258236));
#35964=CARTESIAN_POINT('Ctrl Pts',(3.60300821559048,2.32885918759836,36.2716625040733));
#35965=CARTESIAN_POINT('Ctrl Pts',(3.93054449524549,0.509825557930273,36.1797582617771));
#35966=CARTESIAN_POINT('Ctrl Pts',(3.92785313095816,0.00233337176097839,
36.1541649989355));
#35967=CARTESIAN_POINT('Ctrl Pts',(-2.28358776666034,3.20569428094324,6.5881335146371));
#35968=CARTESIAN_POINT('Ctrl Pts',(-3.35286492248133,2.44407649255814,6.65448899198165));
#35969=CARTESIAN_POINT('Ctrl Pts',(-4.64957922564859,-0.219617924792526,
6.78715544878067));
#35970=CARTESIAN_POINT('Ctrl Pts',(-2.32229699647965,-4.03879127370882,
6.98613288503415));
#35971=CARTESIAN_POINT('Ctrl Pts',(2.14152197144423,-4.13253673306908,7.18506582339759));
#35972=CARTESIAN_POINT('Ctrl Pts',(4.6354962344389,-0.433054729749735,7.38399876176103));
#35973=CARTESIAN_POINT('Ctrl Pts',(2.86863005376323,3.66754880853003,7.58293170012447));
#35974=CARTESIAN_POINT('Ctrl Pts',(-1.53568971473972,4.39499028421212,7.7818646384879));
#35975=CARTESIAN_POINT('Ctrl Pts',(-4.52808181481838,1.08291459320159,7.98079757685135));
#35976=CARTESIAN_POINT('Ctrl Pts',(-3.35787183100746,-3.22511561142074,
8.17973051521478));
#35977=CARTESIAN_POINT('Ctrl Pts',(0.899288778474051,-4.56806013476469,
8.37866345357823));
#35978=CARTESIAN_POINT('Ctrl Pts',(4.32970627742076,-1.7116822031998,8.57759639194166));
#35979=CARTESIAN_POINT('Ctrl Pts',(3.77981709720475,2.71831339521054,8.77652933030509));
#35980=CARTESIAN_POINT('Ctrl Pts',(-0.244881287865563,4.64931963845551,
8.97546226866854));
#35981=CARTESIAN_POINT('Ctrl Pts',(-4.04445595226873,2.30620171359066,9.17439520703196));
#35982=CARTESIAN_POINT('Ctrl Pts',(-4.12594562258144,-2.15702647441609,
9.37332814539542));
#35983=CARTESIAN_POINT('Ctrl Pts',(-0.414433902178747,-4.63728597633392,
9.57226108375884));
#35984=CARTESIAN_POINT('Ctrl Pts',(3.6780683225737,-2.85446979798575,9.77119402212229));
#35985=CARTESIAN_POINT('Ctrl Pts',(4.38930591019076,1.55247461807464,9.97012696048572));
#35986=CARTESIAN_POINT('Ctrl Pts',(1.06543455816436,4.53222144777138,10.1690598988492));
#35987=CARTESIAN_POINT('Ctrl Pts',(-3.23789554621589,3.34547689252468,10.3679928372126));
#35988=CARTESIAN_POINT('Ctrl Pts',(-4.56461363563294,-0.916779903504382,
10.566925775576));
#35989=CARTESIAN_POINT('Ctrl Pts',(-1.69506170633405,-4.33623668960493,
10.7658587139395));
#35990=CARTESIAN_POINT('Ctrl Pts',(2.73276812195122,-3.76937148311671,10.9647916523029));
#35991=CARTESIAN_POINT('Ctrl Pts',(4.64835183630865,0.262694034166192,11.1637245906663));
#35992=CARTESIAN_POINT('Ctrl Pts',(2.29068463981999,4.05326372260543,11.3626575290298));
#35993=CARTESIAN_POINT('Ctrl Pts',(-2.17281932557235,4.11764970909905,11.5615904673932));
#35994=CARTESIAN_POINT('Ctrl Pts',(-4.63884063895772,0.396661654349383,
11.7605234057567));
#35995=CARTESIAN_POINT('Ctrl Pts',(-2.84035473048496,-3.68897925500734,
11.9594563441201));
#35996=CARTESIAN_POINT('Ctrl Pts',(1.56928215333904,-4.38332481861607,12.1583892824835));
#35997=CARTESIAN_POINT('Ctrl Pts',(4.53627084208731,-1.04806001180736,12.357322220847));
#35998=CARTESIAN_POINT('Ctrl Pts',(3.33304518836854,3.25069111315414,12.5562551592104));
#35999=CARTESIAN_POINT('Ctrl Pts',(-0.934264011548026,4.56106716657885,
12.7551880975738));
#36000=CARTESIAN_POINT('Ctrl Pts',(-4.34270007180307,1.67843350404123,12.9541210359373));
#36001=CARTESIAN_POINT('Ctrl Pts',(-3.75887227597289,-2.74719168498093,
13.1530539743007));
#36002=CARTESIAN_POINT('Ctrl Pts',(0.280503837458128,-4.6473111084089,13.3519869126642));
#36003=CARTESIAN_POINT('Ctrl Pts',(4.0620115019401,-2.27513636937342,13.5509198510276));
#36004=CARTESIAN_POINT('Ctrl Pts',(4.10929358463094,2.18858154439125,13.749852789391));
#36005=CARTESIAN_POINT('Ctrl Pts',(0.378883452643525,4.64032652627596,13.9487857277545));
#36006=CARTESIAN_POINT('Ctrl Pts',(-3.6998359543678,2.82619830371296,14.1477186661179));
#36007=CARTESIAN_POINT('Ctrl Pts',(-4.37727940176434,-1.5860668271018,14.3466516044813));
#36008=CARTESIAN_POINT('Ctrl Pts',(-1.03067005834432,-4.54025353608988,
14.5455845428448));
#36009=CARTESIAN_POINT('Ctrl Pts',(3.26343894045982,-3.32056459401619,14.7445174812082));
#36010=CARTESIAN_POINT('Ctrl Pts',(4.55745373218093,0.951734427334463,14.9434504195717));
#36011=CARTESIAN_POINT('Ctrl Pts',(1.66178065462684,4.34909967660568,15.1423833579351));
#36012=CARTESIAN_POINT('Ctrl Pts',(-2.7615749095149,3.74831788410233,15.3413162962985));
#36013=CARTESIAN_POINT('Ctrl Pts',(-4.64620214454805,-0.298309525729033,
15.540249234662));
#36014=CARTESIAN_POINT('Ctrl Pts',(-2.25955469263049,-4.07069963669087,
15.7391821730254));
#36015=CARTESIAN_POINT('Ctrl Pts',(2.20431162797926,-4.10087712421368,15.9381151113889));
#36016=CARTESIAN_POINT('Ctrl Pts',(4.64174427957893,-0.361099687260673,
16.1370480497523));
#36017=CARTESIAN_POINT('Ctrl Pts',(2.81200037969602,3.71063832860775,16.3359809881157));
#36018=CARTESIAN_POINT('Ctrl Pts',(-1.60282821254903,4.37116971326904,16.5349139264792));
#36019=CARTESIAN_POINT('Ctrl Pts',(-4.54416956536685,1.01326497143505,16.7338468648426));
#36020=CARTESIAN_POINT('Ctrl Pts',(-3.30803524366227,-3.27613885051165,
16.932779803206));
#36021=CARTESIAN_POINT('Ctrl Pts',(0.969190868759014,-4.55377338051179,
17.1317127415695));
#36022=CARTESIAN_POINT('Ctrl Pts',(4.35543542339085,-1.6451034052046,17.3306456799329));
#36023=CARTESIAN_POINT('Ctrl Pts',(3.73770845551644,2.77591758571908,17.5295786182963));
#36024=CARTESIAN_POINT('Ctrl Pts',(-0.316110833907594,4.64502496030214,
17.7285115566598));
#36025=CARTESIAN_POINT('Ctrl Pts',(-4.07932800118232,2.24393983874646,17.9274444950232));
#36026=CARTESIAN_POINT('Ctrl Pts',(-4.09240045043936,-2.22000934556306,
18.1263774333867));
#36027=CARTESIAN_POINT('Ctrl Pts',(-0.343310619835542,-4.64309387794946,
18.3253103717501));
#36028=CARTESIAN_POINT('Ctrl Pts',(3.72138621938403,-2.79776116695515,18.5242433101136));
#36029=CARTESIAN_POINT('Ctrl Pts',(4.36499584269893,1.61956606359996,18.723176248477));
#36030=CARTESIAN_POINT('Ctrl Pts',(0.995845006712163,4.54801887240478,18.9221091868404));
#36031=CARTESIAN_POINT('Ctrl Pts',(-3.28879065687452,3.29545732128312,19.1210421252039));
#36032=CARTESIAN_POINT('Ctrl Pts',(-4.55002616559029,-0.986633079511998,
19.3199750635673));
#36033=CARTESIAN_POINT('Ctrl Pts',(-1.62840200065756,-4.36170721912855,
19.5189080019307));
#36034=CARTESIAN_POINT('Ctrl Pts',(2.79021950300484,-3.72704414599493,19.7178409402942));
#36035=CARTESIAN_POINT('Ctrl Pts',(4.64377957295296,0.333907500617121,19.9167738786576));
#36036=CARTESIAN_POINT('Ctrl Pts',(2.22829203699626,4.08789646872357,20.115706817021));
#36037=CARTESIAN_POINT('Ctrl Pts',(-2.23567446665327,4.08386368777145,20.3146397553845));
#36038=CARTESIAN_POINT('Ctrl Pts',(-4.6443753015709,0.325516511565617,20.5135726937479));
#36039=CARTESIAN_POINT('Ctrl Pts',(-2.78348087456552,-3.73207946888481,
20.7125056321114));
#36040=CARTESIAN_POINT('Ctrl Pts',(1.63628013449202,-4.35875788070528,20.9114385704748));
#36041=CARTESIAN_POINT('Ctrl Pts',(4.55180140068407,-0.978410419953773,
21.1103715088382));
#36042=CARTESIAN_POINT('Ctrl Pts',(3.28283101156097,3.30139417378129,21.3093044472017));
#36043=CARTESIAN_POINT('Ctrl Pts',(-1.00406080348858,4.54621214243697,21.5082373855651));
#36044=CARTESIAN_POINT('Ctrl Pts',(-4.36791497172966,1.61167668621328,21.7071703239285));
#36045=CARTESIAN_POINT('Ctrl Pts',(-3.71632511212236,-2.80448045137639,
21.906103262292));
#36046=CARTESIAN_POINT('Ctrl Pts',(0.351699264548243,-4.64246600078663,
22.1050362006554));
#36047=CARTESIAN_POINT('Ctrl Pts',(4.0964049135034,-2.21261151713735,22.3039691390189));
#36048=CARTESIAN_POINT('Ctrl Pts',(4.07526696155566,2.25130676123813,22.5029020773823));
#36049=CARTESIAN_POINT('Ctrl Pts',(0.307717623722685,4.64558853162805,22.7018350157458));
#36050=CARTESIAN_POINT('Ctrl Pts',(-3.74271792010062,2.76915971220537,22.9007679541091));
#36051=CARTESIAN_POINT('Ctrl Pts',(-4.35245591888036,-1.65297017981175,
23.0997008924726));
#36052=CARTESIAN_POINT('Ctrl Pts',(-0.96096146715276,-4.55551709466568,
23.298633830836));
#36053=CARTESIAN_POINT('Ctrl Pts',(3.31394921617401,-3.27015649988854,23.4975667691995));
#36054=CARTESIAN_POINT('Ctrl Pts',(4.54233136705332,1.02147378479679,23.6964997075629));
#36055=CARTESIAN_POINT('Ctrl Pts',(1.59492770745015,4.37405859004556,23.8954326459263));
#36056=CARTESIAN_POINT('Ctrl Pts',(-2.8187002214397,3.70555151128673,24.0943655842898));
#36057=CARTESIAN_POINT('Ctrl Pts',(-4.64108426309036,-0.369485864463859,
24.2932985226532));
#36058=CARTESIAN_POINT('Ctrl Pts',(-2.19689850940736,-4.10485321059198,
24.4922314610167));
#36059=CARTESIAN_POINT('Ctrl Pts',(2.26690599978809,-4.06661039801803,24.6911643993801));
#36060=CARTESIAN_POINT('Ctrl Pts',(4.64673355030702,-0.289914217648445,
24.8900973377435));
#36061=CARTESIAN_POINT('Ctrl Pts',(2.75479789015282,3.75330141682668,25.089030276107));
#36062=CARTESIAN_POINT('Ctrl Pts',(-1.66963595449858,4.34609004975612,25.2879632144704));
#36063=CARTESIAN_POINT('Ctrl Pts',(-4.55916589979193,0.943498404512721,
25.4868961528339));
#36064=CARTESIAN_POINT('Ctrl Pts',(-3.25743397236614,-3.32645559970645,
25.6858290911973));
#36065=CARTESIAN_POINT('Ctrl Pts',(1.03887176776102,-4.5383838964209,25.8847620295608));
#36066=CARTESIAN_POINT('Ctrl Pts',(4.38013798386919,-1.57815531029427,26.0836949679242));
#36067=CARTESIAN_POINT('Ctrl Pts',(3.69472350167733,2.8328786044052,26.2826279062876));
#36068=CARTESIAN_POINT('Ctrl Pts',(-0.387267039202406,4.63963438015227,
26.4815608446511));
#36069=CARTESIAN_POINT('Ctrl Pts',(-4.11324123594255,2.18115324452121,26.6804937830145));
#36070=CARTESIAN_POINT('Ctrl Pts',(-4.05789412426333,-2.28247195325872,
26.8794267213779));
#36071=CARTESIAN_POINT('Ctrl Pts',(-0.272106554751227,-4.64781034079544,
27.0783596597414));
#36072=CARTESIAN_POINT('Ctrl Pts',(3.76382980366497,-2.74039561928326,27.2772925981048));
#36073=CARTESIAN_POINT('Ctrl Pts',(4.33966036680293,1.68627721384812,27.4762255364683));
#36074=CARTESIAN_POINT('Ctrl Pts',(0.926021488444692,4.56274776248724,27.6751584748317));
#36075=CARTESIAN_POINT('Ctrl Pts',(-3.33891314074683,3.24466361579928,27.8740914131951));
#36076=CARTESIAN_POINT('Ctrl Pts',(-4.53436978850062,-1.056254496926,28.0730243515586));
#36077=CARTESIAN_POINT('Ctrl Pts',(-1.56135974101536,-4.38615306393655,
28.271957289922));
#36078=CARTESIAN_POINT('Ctrl Pts',(2.84701539209114,-3.68384124228226,28.4708902282854));
#36079=CARTESIAN_POINT('Ctrl Pts',(4.63811637326107,0.405042527682263,28.6698231666489));
#36080=CARTESIAN_POINT('Ctrl Pts',(2.16537595366717,4.12156886639343,28.8687561050123));
#36081=CARTESIAN_POINT('Ctrl Pts',(-2.29800439309459,4.04911826827293,29.0676890433758));
#36082=CARTESIAN_POINT('Ctrl Pts',(-4.64881888728275,0.254294896501576,
29.2666219817392));
#36083=CARTESIAN_POINT('Ctrl Pts',(-2.72595311106574,-3.77430292602682,
29.4655549201026));
#36084=CARTESIAN_POINT('Ctrl Pts',(1.70289371351612,-4.33316696442807,29.6644878584661));
#36085=CARTESIAN_POINT('Ctrl Pts',(4.56626263015895,-0.908530975562921,
29.8634207968295));
#36086=CARTESIAN_POINT('Ctrl Pts',(3.23184561769564,3.35132165638052,30.0623537351929));
#36087=CARTESIAN_POINT('Ctrl Pts',(-1.07362171706024,4.53028910223179,30.2612866735564));
#36088=CARTESIAN_POINT('Ctrl Pts',(-4.39210374192795,1.54454124622366,30.4602196119198));
#36089=CARTESIAN_POINT('Ctrl Pts',(-3.67290489288628,-2.86111037692635,
30.6591525502832));
#36090=CARTESIAN_POINT('Ctrl Pts',(0.422812068905003,-4.63653026470569,
30.8580854886467));
#36091=CARTESIAN_POINT('Ctrl Pts',(4.12983597966957,-2.14956686850405,31.0570184270101));
#36092=CARTESIAN_POINT('Ctrl Pts',(4.04028295890316,2.31350309123207,31.2559513653736));
#36093=CARTESIAN_POINT('Ctrl Pts',(0.236479504429024,4.64975917496042,31.454884303737));
#36094=CARTESIAN_POINT('Ctrl Pts',(-3.78472063013482,2.71147057756036,31.6538172421005));
#36095=CARTESIAN_POINT('Ctrl Pts',(-4.32660993797449,-1.71948520952171,
31.8527501804639));
#36096=CARTESIAN_POINT('Ctrl Pts',(-0.891027122681378,-4.56971045119814,
32.0516831188273));
#36097=CARTESIAN_POINT('Ctrl Pts',(3.36368096441276,-3.21898016626241,32.2506160571907));
#36098=CARTESIAN_POINT('Ctrl Pts',(4.5261418975313,1.09097317316021,32.4495489955542));
#36099=CARTESIAN_POINT('Ctrl Pts',(1.52770007286572,4.39798993046933,32.6484819339176));
#36100=CARTESIAN_POINT('Ctrl Pts',(-2.87516335195365,3.66191461406821,32.8474148722811));
#36101=CARTESIAN_POINT('Ctrl Pts',(-4.63487607777506,-0.4405754019598,33.0463478106445));
#36102=CARTESIAN_POINT('Ctrl Pts',(-2.13372622115719,-4.13804245438466,
33.245280749008));
#36103=CARTESIAN_POINT('Ctrl Pts',(2.3289678201032,-4.03138832588321,33.4442136873714));
#36104=CARTESIAN_POINT('Ctrl Pts',(4.65063119002216,-0.218660640117578,
33.6431466257348));
#36105=CARTESIAN_POINT('Ctrl Pts',(2.69694823141472,3.79508276302539,33.8420795640982));
#36106=CARTESIAN_POINT('Ctrl Pts',(-1.73605145825132,4.31998938371931,34.0410125024617));
#36107=CARTESIAN_POINT('Ctrl Pts',(-4.57309117498029,0.873510186809756,
34.2399454408251));
#36108=CARTESIAN_POINT('Ctrl Pts',(-3.20606745040362,-3.37599088337116,
34.4388783791886));
#36109=CARTESIAN_POINT('Ctrl Pts',(1.10830861045392,-4.52192823529311,34.637811317552));
#36110=CARTESIAN_POINT('Ctrl Pts',(4.4038115431333,-1.51083646822047,34.8367442559154));
#36111=CARTESIAN_POINT('Ctrl Pts',(3.65087056719927,2.88917411083122,35.0356771942789));
#36112=CARTESIAN_POINT('Ctrl Pts',(-0.458332266027874,4.63315383676036,
35.2346101326423));
#36113=CARTESIAN_POINT('Ctrl Pts',(-4.1461881700408,2.11785424421031,35.4335430710058));
#36114=CARTESIAN_POINT('Ctrl Pts',(-4.02243449981698,-2.3443983526288,35.6324760093692));
#36115=CARTESIAN_POINT('Ctrl Pts',(-0.200838565195405,-4.65143491968315,
35.8314089477326));
#36116=CARTESIAN_POINT('Ctrl Pts',(3.80538917253758,-2.68238628582457,36.0303418860961));
#36117=CARTESIAN_POINT('Ctrl Pts',(4.313305398898,1.75259221639213,36.2292748244595));
#36118=CARTESIAN_POINT('Ctrl Pts',(0.855980425100957,4.57640475199999,36.428207762823));
#36119=CARTESIAN_POINT('Ctrl Pts',(-3.3882512324144,3.19310765946044,36.6271407011864));
#36120=CARTESIAN_POINT('Ctrl Pts',(-4.51764817756711,-1.1256277739117,36.8260736395498));
#36121=CARTESIAN_POINT('Ctrl Pts',(-1.49395067955099,-4.40956849538517,
37.0250065779133));
#36122=CARTESIAN_POINT('Ctrl Pts',(2.90314244717482,-3.63977291262905,37.2239395162767));
#36123=CARTESIAN_POINT('Ctrl Pts',(4.63136356822164,0.476082396912402,37.4228724546401));
#36124=CARTESIAN_POINT('Ctrl Pts',(2.10195116827292,4.15427301369114,37.6218053930036));
#36125=CARTESIAN_POINT('Ctrl Pts',(-2.35979445756394,4.01342159940947,37.820738331367));
#36126=CARTESIAN_POINT('Ctrl Pts',(-4.6521703611112,0.183013565819844,38.0196712697305));
#36127=CARTESIAN_POINT('Ctrl Pts',(-2.66778493740627,-3.81563975427051,
38.2186042080939));
#36128=CARTESIAN_POINT('Ctrl Pts',(1.76910720810075,-4.30655799166989,38.4175371464573));
#36129=CARTESIAN_POINT('Ctrl Pts',(4.57965119683031,-0.838438267478442,
38.6164700848208));
#36130=CARTESIAN_POINT('Ctrl Pts',(3.18010086249031,3.40046216234224,38.8154030231842));
#36131=CARTESIAN_POINT('Ctrl Pts',(-1.14293017678358,4.51330115287866,39.0143359615477));
#36132=CARTESIAN_POINT('Ctrl Pts',(-4.4152611484038,1.47704417104799,39.2132688999111));
#36133=CARTESIAN_POINT('Ctrl Pts',(-3.6286209586944,-2.91707048796121,39.4122018382745));
#36134=CARTESIAN_POINT('Ctrl Pts',(0.493823895339948,-4.62950082687821,
39.6111347766379));
#36135=CARTESIAN_POINT('Ctrl Pts',(4.16230000860224,-2.08602580072547,39.8100677150015));
#36136=CARTESIAN_POINT('Ctrl Pts',(4.00434373250677,2.37517234857208,40.0090006533648));
#36137=CARTESIAN_POINT('Ctrl Pts',(0.16519745519922,4.6528059816321,40.2079335917283));
#36138=CARTESIAN_POINT('Ctrl Pts',(-3.82585650677666,2.65320484133016,40.4068665300917));
#36139=CARTESIAN_POINT('Ctrl Pts',(-4.29970479193952,-1.78571208206424,
40.6057994684551));
#36140=CARTESIAN_POINT('Ctrl Pts',(-0.820965403692237,-4.58260824249866,
40.8047324068186));
#36141=CARTESIAN_POINT('Ctrl Pts',(3.41277964200003,-3.16747340374845,41.003665345182));
#36142=CARTESIAN_POINT('Ctrl Pts',(4.50858774680517,1.16103327592888,41.2025982835454));
#36143=CARTESIAN_POINT('Ctrl Pts',(1.46069211445911,4.41931609540443,41.4015312219089));
#36144=CARTESIAN_POINT('Ctrl Pts',(-2.93206675809147,3.62048102032587,41.6004641602723));
#36145=CARTESIAN_POINT('Ctrl Pts',(-4.62538118106894,-0.517884424352666,
41.7993970986358));
#36146=CARTESIAN_POINT('Ctrl Pts',(-2.92506802252003,-2.94215747695014,
41.9320190575447));
#36147=CARTESIAN_POINT('Ctrl Pts',(-1.74998052418886,-3.52545282590189,
41.9983300369992));
#36148=CARTESIAN_POINT('Ctrl Pts',(-2.14454317821952,3.01050386677641,6.72649619915742));
#36149=CARTESIAN_POINT('Ctrl Pts',(-3.14871348584711,2.29525996140177,6.79285167650196));
#36150=CARTESIAN_POINT('Ctrl Pts',(-4.36647259874689,-0.206245684665433,
6.92551813330099));
#36151=CARTESIAN_POINT('Ctrl Pts',(-2.18089545508631,-3.7928747038927,7.12449556955447));
#36152=CARTESIAN_POINT('Ctrl Pts',(2.01112757824255,-3.88091212828921,7.32342850791792));
#36153=CARTESIAN_POINT('Ctrl Pts',(4.35324710193498,-0.406686609570857,
7.52236144628135));
#36154=CARTESIAN_POINT('Ctrl Pts',(2.69396302714936,3.44423669322017,7.7212943846448));
#36155=CARTESIAN_POINT('Ctrl Pts',(-1.44218363300452,4.12738523561646,7.92022732300823));
#36156=CARTESIAN_POINT('Ctrl Pts',(-4.25237300188823,1.01697737978396,8.11916026137167));
#36157=CARTESIAN_POINT('Ctrl Pts',(-3.15341553044576,-3.02874265855638,
8.31809319973511));
#36158=CARTESIAN_POINT('Ctrl Pts',(0.844532293999059,-4.28991709569067,
8.51702613809854));
#36159=CARTESIAN_POINT('Ctrl Pts',(4.06607628421319,-1.60746017549409,8.71595907646199));
#36160=CARTESIAN_POINT('Ctrl Pts',(3.54966911676128,2.55279894780965,8.91489201482541));
#36161=CARTESIAN_POINT('Ctrl Pts',(-0.229970795531832,4.36622881746894,
9.11382495318887));
#36162=CARTESIAN_POINT('Ctrl Pts',(-3.79819446779221,2.16578019232958,9.31275789155229));
#36163=CARTESIAN_POINT('Ctrl Pts',(-3.87472234165631,-2.02568803287688,
9.51169082991574));
#36164=CARTESIAN_POINT('Ctrl Pts',(-0.389199579151803,-4.35492786885263,
9.71062376827917));
#36165=CARTESIAN_POINT('Ctrl Pts',(3.45411568819898,-2.6806649703053,9.90955670664261));
#36166=CARTESIAN_POINT('Ctrl Pts',(4.12204697548566,1.45794652614552,10.1084896450061));
#36167=CARTESIAN_POINT('Ctrl Pts',(1.00056168057528,4.25626057815718,10.3074225833695));
#36168=CARTESIAN_POINT('Ctrl Pts',(-3.04074444030663,3.14177530310008,10.5063555217329));
#36169=CARTESIAN_POINT('Ctrl Pts',(-4.28668044925664,-0.860958407946073,
10.7052884600964));
#36170=CARTESIAN_POINT('Ctrl Pts',(-1.59185167833342,-4.07220906838072,
10.9042213984598));
#36171=CARTESIAN_POINT('Ctrl Pts',(2.56637354567592,-3.53985952206916,11.1031543368232));
#36172=CARTESIAN_POINT('Ctrl Pts',(4.36531994349343,0.246698947662476,11.3020872751867));
#36173=CARTESIAN_POINT('Ctrl Pts',(2.15120793231547,3.80646594483665,11.5010202135501));
#36174=CARTESIAN_POINT('Ctrl Pts',(-2.04051927856241,3.86693155519059,11.6999531519136));
#36175=CARTESIAN_POINT('Ctrl Pts',(-4.35638787015977,0.372509459594964,
11.898886090277));
#36176=CARTESIAN_POINT('Ctrl Pts',(-2.66740935028452,-3.46436226862834,
12.0978190286404));
#36177=CARTESIAN_POINT('Ctrl Pts',(1.47373067318826,-4.11643006453438,12.2967519670039));
#36178=CARTESIAN_POINT('Ctrl Pts',(4.2600634102983,-0.984245046982922,12.4956849053673));
#36179=CARTESIAN_POINT('Ctrl Pts',(3.13010054869347,3.05276090237982,12.6946178437308));
#36180=CARTESIAN_POINT('Ctrl Pts',(-0.877377932161288,4.28334991993443,
12.8935507820942));
#36181=CARTESIAN_POINT('Ctrl Pts',(-4.07827890392793,1.57623594491877,13.0924837204576));
#36182=CARTESIAN_POINT('Ctrl Pts',(-3.52999959753036,-2.57991887734767,
13.2914166588211));
#36183=CARTESIAN_POINT('Ctrl Pts',(0.263424335980266,-4.36434258411605,
13.4903495971845));
#36184=CARTESIAN_POINT('Ctrl Pts',(3.8146810836505,-2.1366063751491,13.6892825355479));
#36185=CARTESIAN_POINT('Ctrl Pts',(3.85908422390511,2.05532175707241,13.8882154739114));
#36186=CARTESIAN_POINT('Ctrl Pts',(0.355813748685168,4.35778328379722,14.0871484122748));
#36187=CARTESIAN_POINT('Ctrl Pts',(-3.47455791816341,2.65411488930297,14.2860813506383));
#36188=CARTESIAN_POINT('Ctrl Pts',(-4.11075274498564,-1.48949335073545,
14.4850142890017));
#36189=CARTESIAN_POINT('Ctrl Pts',(-0.967913944402505,-4.26380360341846,
14.6839472273652));
#36190=CARTESIAN_POINT('Ctrl Pts',(3.06473253162247,-3.11837988094897,14.8828801657286));
#36191=CARTESIAN_POINT('Ctrl Pts',(4.27995650269812,0.893784597822432,15.081813104092));
#36192=CARTESIAN_POINT('Ctrl Pts',(1.56059706511263,4.08428884539946,15.2807460424554));
#36193=CARTESIAN_POINT('Ctrl Pts',(-2.59342632668046,3.52008784838862,15.4796789808189));
#36194=CARTESIAN_POINT('Ctrl Pts',(-4.3633011435735,-0.280145859835127,
15.6786119191823));
#36195=CARTESIAN_POINT('Ctrl Pts',(-2.12197344575085,-3.82284020955897,
15.8775448575457));
#36196=CARTESIAN_POINT('Ctrl Pts',(2.0700940570225,-3.8511802304453,16.0764777959092));
#36197=CARTESIAN_POINT('Ctrl Pts',(4.35911471200799,-0.339112812863191,
16.2754107342726));
#36198=CARTESIAN_POINT('Ctrl Pts',(2.6407814577879,3.48470255036153,16.4743436726361));
#36199=CARTESIAN_POINT('Ctrl Pts',(-1.50523415796133,4.10501506720731,16.6732766109995));
#36200=CARTESIAN_POINT('Ctrl Pts',(-4.26748119093852,0.951568629831059,
16.8722095493629));
#36201=CARTESIAN_POINT('Ctrl Pts',(-3.10661342589027,-3.07665916122845,
17.0711424877264));
#36202=CARTESIAN_POINT('Ctrl Pts',(0.910178140001792,-4.27650024269325,
17.2700754260898));
#36203=CARTESIAN_POINT('Ctrl Pts',(4.09023881708235,-1.54493527098234,17.4690083644533));
#36204=CARTESIAN_POINT('Ctrl Pts',(3.51012441364316,2.60689569661673,17.6679413028167));
#36205=CARTESIAN_POINT('Ctrl Pts',(-0.296863270295577,4.36219563649339,
17.8668742411801));
#36206=CARTESIAN_POINT('Ctrl Pts',(-3.83094320453884,2.10730935932299,18.0658071795436));
#36207=CARTESIAN_POINT('Ctrl Pts',(-3.84321968993877,-2.08483596169087,
18.264740117907));
#36208=CARTESIAN_POINT('Ctrl Pts',(-0.322406897833154,-4.3603821351485,
18.4636730562704));
#36209=CARTESIAN_POINT('Ctrl Pts',(3.4947960165208,-2.62740925156378,18.6626059946339));
#36210=CARTESIAN_POINT('Ctrl Pts',(4.09921711531441,1.52095286376864,18.8615389329973));
#36211=CARTESIAN_POINT('Ctrl Pts',(0.935209343336036,4.27109611884696,19.0604718713608));
#36212=CARTESIAN_POINT('Ctrl Pts',(-3.08854061611436,3.09480135629163,19.2594048097242));
#36213=CARTESIAN_POINT('Ctrl Pts',(-4.27298119064957,-0.926558317996034,
19.4583377480876));
#36214=CARTESIAN_POINT('Ctrl Pts',(-1.52925079250028,-4.09612873161108,
19.6572706864511));
#36215=CARTESIAN_POINT('Ctrl Pts',(2.62032678939031,-3.50010943958843,19.8562036248145));
#36216=CARTESIAN_POINT('Ctrl Pts',(4.36102607910528,0.313576321899792,20.055136563178));
#36217=CARTESIAN_POINT('Ctrl Pts',(2.09261433118024,3.83898994961327,20.2540695015414));
#36218=CARTESIAN_POINT('Ctrl Pts',(-2.09954725462231,3.83520271927058,20.4530024399048));
#36219=CARTESIAN_POINT('Ctrl Pts',(-4.36158553460872,0.30569624888859,20.6519353782683));
#36220=CARTESIAN_POINT('Ctrl Pts',(-2.61399846697548,-3.50483816843836,
20.8508683166317));
#36221=CARTESIAN_POINT('Ctrl Pts',(1.53664923735901,-4.09335897443855,21.0498012549951));
#36222=CARTESIAN_POINT('Ctrl Pts',(4.27464833406557,-0.918836325121606,
21.2487341933586));
#36223=CARTESIAN_POINT('Ctrl Pts',(3.08294384559025,3.10037672182424,21.447667131722));
#36224=CARTESIAN_POINT('Ctrl Pts',(-0.942924891294206,4.26939939823746,
21.6466000700854));
#36225=CARTESIAN_POINT('Ctrl Pts',(-4.10195850250371,1.51354385996249,21.8455330084489));
#36226=CARTESIAN_POINT('Ctrl Pts',(-3.49004307327481,-2.63371940779178,
22.0444659468123));
#36227=CARTESIAN_POINT('Ctrl Pts',(0.330284769249194,-4.35979248858183,
22.2433988851758));
#36228=CARTESIAN_POINT('Ctrl Pts',(3.84698032663149,-2.07788857709042,22.4423318235392));
#36229=CARTESIAN_POINT('Ctrl Pts',(3.82712943615432,2.11422771981017,22.6412647619026));
#36230=CARTESIAN_POINT('Ctrl Pts',(0.288981111392786,4.36272489271909,22.8401977002661));
#36231=CARTESIAN_POINT('Ctrl Pts',(-3.51482885866484,2.6005493009342,23.0391306386295));
#36232=CARTESIAN_POINT('Ctrl Pts',(-4.08744073059509,-1.5523230482618,23.238063576993));
#36233=CARTESIAN_POINT('Ctrl Pts',(-0.902449815593572,-4.27813778443702,
23.4369965153564));
#36234=CARTESIAN_POINT('Ctrl Pts',(3.11216730456806,-3.07104106789052,23.6359294537198));
#36235=CARTESIAN_POINT('Ctrl Pts',(4.26575491804855,0.959277619585273,23.8348623920833));
#36236=CARTESIAN_POINT('Ctrl Pts',(1.4978147039944,4.10772804416148,24.0337953304467));
#36237=CARTESIAN_POINT('Ctrl Pts',(-2.64707335517684,3.47992546250712,24.2327282688101));
#36238=CARTESIAN_POINT('Ctrl Pts',(-4.35849488303591,-0.346988367013049,
24.4316612071736));
#36239=CARTESIAN_POINT('Ctrl Pts',(-2.06313231327231,-3.85491421827051,
24.630594145537));
#36240=CARTESIAN_POINT('Ctrl Pts',(2.12887714170064,-3.81899995913029,24.8295270839005));
#36241=CARTESIAN_POINT('Ctrl Pts',(4.36380019275037,-0.272261730774709,
25.0284600222639));
#36242=CARTESIAN_POINT('Ctrl Pts',(2.58706195091454,3.52476794050656,25.2273929606274));
#36243=CARTESIAN_POINT('Ctrl Pts',(-1.56797406633792,4.08146247068183,25.4263258989908));
#36244=CARTESIAN_POINT('Ctrl Pts',(-4.28156441872558,0.886050055355632,
25.6252588373542));
#36245=CARTESIAN_POINT('Ctrl Pts',(-3.05909319796137,-3.12391219122417,
25.8241917757177));
#36246=CARTESIAN_POINT('Ctrl Pts',(0.975616262761357,-4.2620478035949,26.0231247140811));
#36247=CARTESIAN_POINT('Ctrl Pts',(4.11343727186996,-1.48206355554802,26.2220576524445));
#36248=CARTESIAN_POINT('Ctrl Pts',(3.46975675584276,2.6603884354688,26.4209905908079));
#36249=CARTESIAN_POINT('Ctrl Pts',(-0.363686869931574,4.35713328152031,
26.6199235291714));
#36250=CARTESIAN_POINT('Ctrl Pts',(-3.86279150803662,2.0483457563929,26.8188564675348));
#36251=CARTESIAN_POINT('Ctrl Pts',(-3.810814407564,-2.14349530519553,27.0177894058983));
#36252=CARTESIAN_POINT('Ctrl Pts',(-0.255538352525876,-4.36481141891387,
27.2167223442617));
#36253=CARTESIAN_POINT('Ctrl Pts',(3.53465526802747,-2.57353661495193,27.4156552826252));
#36254=CARTESIAN_POINT('Ctrl Pts',(4.07542428247787,1.58360206178266,27.6145882209886));
#36255=CARTESIAN_POINT('Ctrl Pts',(0.869637285206309,4.28492818661779,27.813521159352));
#36256=CARTESIAN_POINT('Ctrl Pts',(-3.13561120934189,3.04710041123396,28.0124540977155));
#36257=CARTESIAN_POINT('Ctrl Pts',(-4.25827810930823,-0.99194058092151,
28.2113870360789));
#36258=CARTESIAN_POINT('Ctrl Pts',(-1.46629064589802,-4.11908610180032,
28.4103199744424));
#36259=CARTESIAN_POINT('Ctrl Pts',(2.67366445316185,-3.4595371025892,28.6092529128058));
#36260=CARTESIAN_POINT('Ctrl Pts',(4.35570770402749,0.380380032820054,28.8081858511692));
#36261=CARTESIAN_POINT('Ctrl Pts',(2.03352912356371,3.87061208026725,29.0071187895327));
#36262=CARTESIAN_POINT('Ctrl Pts',(-2.15808199565578,3.80257290164423,29.2060517278961));
#36263=CARTESIAN_POINT('Ctrl Pts',(-4.36575855636173,0.238811222196252,
29.4049846662595));
#36264=CARTESIAN_POINT('Ctrl Pts',(-2.55997349163937,-3.5444906960516,29.603917604623));
#36265=CARTESIAN_POINT('Ctrl Pts',(1.59920680512957,-4.06932625464213,29.8028505429864));
#36266=CARTESIAN_POINT('Ctrl Pts',(4.2882290387233,-0.853211746134946,30.0017834813498));
#36267=CARTESIAN_POINT('Ctrl Pts',(3.03506288379887,3.14726418714398,30.2007164197133));
#36268=CARTESIAN_POINT('Ctrl Pts',(-1.00825033437494,4.25444589053914,30.3996493580767));
#36269=CARTESIAN_POINT('Ctrl Pts',(-4.12467445101052,1.45049620663885,30.5985822964402));
#36270=CARTESIAN_POINT('Ctrl Pts',(-3.44926665280217,-2.68690121332354,
30.7975152348036));
#36271=CARTESIAN_POINT('Ctrl Pts',(0.397067610571902,-4.35421817148927,
30.996448173167));
#36272=CARTESIAN_POINT('Ctrl Pts',(3.87837582013254,-2.01868263233817,31.1953811115305));
#36273=CARTESIAN_POINT('Ctrl Pts',(3.7942755623814,2.17263699890429,31.3943140498939));
#36274=CARTESIAN_POINT('Ctrl Pts',(0.222080585391179,4.36664159118708,31.5932469882574));
#36275=CARTESIAN_POINT('Ctrl Pts',(-3.55427408016482,2.54637278012491,31.7921799266208));
#36276=CARTESIAN_POINT('Ctrl Pts',(-4.06316847671228,-1.61478806725346,
31.9911128649843));
#36277=CARTESIAN_POINT('Ctrl Pts',(-0.836773679318462,-4.2914669265756,
32.1900458033476));
#36278=CARTESIAN_POINT('Ctrl Pts',(3.15887095352933,-3.02298079240363,32.3889787417111));
#36279=CARTESIAN_POINT('Ctrl Pts',(4.25055120355625,1.02454528364496,32.5879116800745));
#36280=CARTESIAN_POINT('Ctrl Pts',(1.43468046968086,4.1302022374466,32.786844618438));
#36281=CARTESIAN_POINT('Ctrl Pts',(-2.70009852159804,3.43894555728302,32.9857775568014));
#36282=CARTESIAN_POINT('Ctrl Pts',(-4.3526647057765,-0.413749358162806,
33.1847104951649));
#36283=CARTESIAN_POINT('Ctrl Pts',(-2.00380650070783,-3.88608261363723,
33.3836434335282));
#36284=CARTESIAN_POINT('Ctrl Pts',(2.18716010122942,-3.7859225116057,33.5825763718918));
#36285=CARTESIAN_POINT('Ctrl Pts',(4.36746051042428,-0.205346687767176,
33.7815093102551));
#36286=CARTESIAN_POINT('Ctrl Pts',(2.53273468010832,3.56400527671735,33.9804422486186));
#36287=CARTESIAN_POINT('Ctrl Pts',(-1.63034561937406,4.05695103910325,34.179375186982));
#36288=CARTESIAN_POINT('Ctrl Pts',(-4.29464180263262,0.820323326117568,
34.3783081253455));
#36289=CARTESIAN_POINT('Ctrl Pts',(-3.01085431445013,-3.17043133807512,
34.5772410637089));
#36290=CARTESIAN_POINT('Ctrl Pts',(1.04082518947229,-4.24659410554575,34.7761740020724));
#36291=CARTESIAN_POINT('Ctrl Pts',(4.1356693799436,-1.41884366724649,34.9751069404358));
#36292=CARTESIAN_POINT('Ctrl Pts',(3.42857396757734,2.7132561842074,35.1740398787992));
#36293=CARTESIAN_POINT('Ctrl Pts',(-0.43042503065489,4.35104732970134,35.3729728171627));
#36294=CARTESIAN_POINT('Ctrl Pts',(-3.89373234762037,1.98890094709468,35.5719057555261));
#36295=CARTESIAN_POINT('Ctrl Pts',(-3.77751387196871,-2.2016510893785,35.7708386938896));
#36296=CARTESIAN_POINT('Ctrl Pts',(-0.188609775022207,-4.36821530206696,
35.969771632253));
#36297=CARTESIAN_POINT('Ctrl Pts',(3.57368414281305,-2.51905939180415,36.1687045706164));
#36298=CARTESIAN_POINT('Ctrl Pts',(4.05067403312995,1.64587923299354,36.3676375089799));
#36299=CARTESIAN_POINT('Ctrl Pts',(0.803860928027483,4.29775362040325,36.5665704473433));
#36300=CARTESIAN_POINT('Ctrl Pts',(-3.18194517095124,2.99868362775086,36.7655033857068));
#36301=CARTESIAN_POINT('Ctrl Pts',(-4.24257465477942,-1.05708981235569,
36.9644363240701));
#36302=CARTESIAN_POINT('Ctrl Pts',(-1.40298603154328,-4.14107579911404,
37.1633692624336));
#36303=CARTESIAN_POINT('Ctrl Pts',(2.72637400733384,-3.41815203427124,37.362302200797));
#36304=CARTESIAN_POINT('Ctrl Pts',(4.34936606820663,0.447094379937924,37.5612351391605));
#36305=CARTESIAN_POINT('Ctrl Pts',(1.97396618806673,3.90132491601227,37.7601680775239));
#36306=CARTESIAN_POINT('Ctrl Pts',(-2.21610974618682,3.76904975494763,37.9591010158874));
#36307=CARTESIAN_POINT('Ctrl Pts',(-4.3689059634554,0.17187011588989,38.1580339542508));
#36308=CARTESIAN_POINT('Ctrl Pts',(-2.50534709985704,-3.5833105804079,38.3569668926142));
#36309=CARTESIAN_POINT('Ctrl Pts',(1.66138864906423,-4.04433746645492,38.5558998309777));
#36310=CARTESIAN_POINT('Ctrl Pts',(4.30080239357324,-0.787386888794196,
38.7548327693411));
#36311=CARTESIAN_POINT('Ctrl Pts',(2.98646879715839,3.19341259377544,38.9537657077046));
#36312=CARTESIAN_POINT('Ctrl Pts',(-1.07333869518271,4.23849231457894,39.152698646068));
#36313=CARTESIAN_POINT('Ctrl Pts',(-4.14642183414512,1.38710893760937,39.3516315844314));
#36314=CARTESIAN_POINT('Ctrl Pts',(-3.40767910781596,-2.73945398844537,
39.5505645227949));
#36315=CARTESIAN_POINT('Ctrl Pts',(0.46375562238267,-4.34761674667882,39.7494974611583));
#36316=CARTESIAN_POINT('Ctrl Pts',(3.90886315799689,-1.9590104947349,39.9484303995218));
#36317=CARTESIAN_POINT('Ctrl Pts',(3.76052462715392,2.23055129808965,40.1473633378851));
#36318=CARTESIAN_POINT('Ctrl Pts',(0.155138804288171,4.36950288189749,40.3462962762487));
#36319=CARTESIAN_POINT('Ctrl Pts',(-3.59290524859212,2.49165476622559,40.545229214612));
#36320=CARTESIAN_POINT('Ctrl Pts',(-4.03790154884084,-1.67698247458014,
40.7441621529755));
#36321=CARTESIAN_POINT('Ctrl Pts',(-0.770977924188701,-4.3035793887071,
40.943095091339));
#36322=CARTESIAN_POINT('Ctrl Pts',(3.20498007865981,-2.97461020739956,41.1420280297023));
#36323=CARTESIAN_POINT('Ctrl Pts',(4.23406590146329,1.09033952096375,41.3409609680659));
#36324=CARTESIAN_POINT('Ctrl Pts',(1.37175253575807,4.15022988087543,41.5398939064291));
#36325=CARTESIAN_POINT('Ctrl Pts',(-2.75353715585242,3.40003479934917,41.7388268447928));
#36326=CARTESIAN_POINT('Ctrl Pts',(-4.34374794056332,-0.486351138137266,
41.9377597831561));
#36327=CARTESIAN_POINT('Ctrl Pts',(-2.74696456387898,-2.76301346440847,
42.0703817420651));
#36328=CARTESIAN_POINT('Ctrl Pts',(-1.64342656321671,-3.3107927439021,42.1366927215196));
#36329=CARTESIAN_POINT('Ctrl Pts',(-2.0054985897787,2.81531345260957,6.86485888367774));
#36330=CARTESIAN_POINT('Ctrl Pts',(-2.94456204921288,2.14644343024538,6.93121436102229));
#36331=CARTESIAN_POINT('Ctrl Pts',(-4.08336597184518,-0.19287344453834,
7.06388081782131));
#36332=CARTESIAN_POINT('Ctrl Pts',(-2.03949391369296,-3.54695813407657,
7.26285825407481));
#36333=CARTESIAN_POINT('Ctrl Pts',(1.88073318504086,-3.62928752350934,7.46179119243823));
#36334=CARTESIAN_POINT('Ctrl Pts',(4.07099796943106,-0.380318489391973,
7.66072413080168));
#36335=CARTESIAN_POINT('Ctrl Pts',(2.51929600053549,3.2209245779103,7.8596570691651));
#36336=CARTESIAN_POINT('Ctrl Pts',(-1.34867755126933,3.85978018702081,8.05859000752856));
#36337=CARTESIAN_POINT('Ctrl Pts',(-3.97666418895809,0.951040166366322,
8.25752294589198));
#36338=CARTESIAN_POINT('Ctrl Pts',(-2.94895922988404,-2.83236970569201,
8.45645588425543));
#36339=CARTESIAN_POINT('Ctrl Pts',(0.789775809524059,-4.01177405661665,
8.65538882261886));
#36340=CARTESIAN_POINT('Ctrl Pts',(3.80244629100563,-1.50323814778838,8.85432176098231));
#36341=CARTESIAN_POINT('Ctrl Pts',(3.31952113631781,2.38728450040875,9.05325469934573));
#36342=CARTESIAN_POINT('Ctrl Pts',(-0.2150603031981,4.08313799648236,9.25218763770918));
#36343=CARTESIAN_POINT('Ctrl Pts',(-3.5519329833157,2.02535867106851,9.45112057607261));
#36344=CARTESIAN_POINT('Ctrl Pts',(-3.62349906073116,-1.89434959133768,
9.65005351443604));
#36345=CARTESIAN_POINT('Ctrl Pts',(-0.363965256124856,-4.07256976137133,
9.84898645279951));
#36346=CARTESIAN_POINT('Ctrl Pts',(3.23016305382427,-2.50686014262486,10.0479193911629));
#36347=CARTESIAN_POINT('Ctrl Pts',(3.85478804078057,1.36341843421643,10.2468523295264));
#36348=CARTESIAN_POINT('Ctrl Pts',(0.93568880298618,3.98029970854296,10.4457852678898));
#36349=CARTESIAN_POINT('Ctrl Pts',(-2.84359333439737,2.9380737136755,10.6447182062533));
#36350=CARTESIAN_POINT('Ctrl Pts',(-4.00874726288035,-0.805136912387771,
10.8436511446167));
#36351=CARTESIAN_POINT('Ctrl Pts',(-1.48864165033278,-3.8081814471565,11.0425840829802));
#36352=CARTESIAN_POINT('Ctrl Pts',(2.39997896940062,-3.31034756102161,11.2415170213436));
#36353=CARTESIAN_POINT('Ctrl Pts',(4.0822880506782,0.23070386115876,11.440449959707));
#36354=CARTESIAN_POINT('Ctrl Pts',(2.01173122481096,3.55966816706786,11.6393828980705));
#36355=CARTESIAN_POINT('Ctrl Pts',(-1.90821923155247,3.61621340128212,11.8383158364339));
#36356=CARTESIAN_POINT('Ctrl Pts',(-4.07393510136182,0.34835726484055,12.0372487747973));
#36357=CARTESIAN_POINT('Ctrl Pts',(-2.49446397008411,-3.23974528224934,
12.2361817131608));
#36358=CARTESIAN_POINT('Ctrl Pts',(1.3781791930375,-3.84953531045267,12.4351146515242));
#36359=CARTESIAN_POINT('Ctrl Pts',(3.98385597850928,-0.920430082158486,
12.6340475898877));
#36360=CARTESIAN_POINT('Ctrl Pts',(2.92715590901843,2.8548306916055,12.8329805282511));
#36361=CARTESIAN_POINT('Ctrl Pts',(-0.820491852774556,4.00563267329001,
13.0319134666145));
#36362=CARTESIAN_POINT('Ctrl Pts',(-3.81385773605278,1.47403838579632,13.230846404978));
#36363=CARTESIAN_POINT('Ctrl Pts',(-3.30112691908783,-2.41264606971442,
13.4297793433414));
#36364=CARTESIAN_POINT('Ctrl Pts',(0.246344834502405,-4.0813740598232,13.6287122817048));
#36365=CARTESIAN_POINT('Ctrl Pts',(3.56735066536092,-1.99807638092479,13.8276452200683));
#36366=CARTESIAN_POINT('Ctrl Pts',(3.60887486317929,1.92206196975356,14.0265781584317));
#36367=CARTESIAN_POINT('Ctrl Pts',(0.332744044726809,4.07524004131849,14.2255110967952));
#36368=CARTESIAN_POINT('Ctrl Pts',(-3.24927988195903,2.48203147489298,14.4244440351586));
#36369=CARTESIAN_POINT('Ctrl Pts',(-3.84422608820695,-1.39291987436911,
14.623376973522));
#36370=CARTESIAN_POINT('Ctrl Pts',(-0.905157830460687,-3.98735367074704,
14.8223099118855));
#36371=CARTESIAN_POINT('Ctrl Pts',(2.86602612278512,-2.91619516788176,15.0212428502489));
#36372=CARTESIAN_POINT('Ctrl Pts',(4.00245927321531,0.835834768310396,15.2201757886123));
#36373=CARTESIAN_POINT('Ctrl Pts',(1.45941347559844,3.81947801419324,15.4191087269758));
#36374=CARTESIAN_POINT('Ctrl Pts',(-2.42527774384603,3.29185781267492,15.6180416653392));
#36375=CARTESIAN_POINT('Ctrl Pts',(-4.08040014259896,-0.261982193941216,
15.8169746037027));
#36376=CARTESIAN_POINT('Ctrl Pts',(-1.98439219887121,-3.57498078242707,
16.0159075420661));
#36377=CARTESIAN_POINT('Ctrl Pts',(1.93587648606574,-3.60148333667693,16.2148404804295));
#36378=CARTESIAN_POINT('Ctrl Pts',(4.07648514443705,-0.317125938465704,
16.413773418793));
#36379=CARTESIAN_POINT('Ctrl Pts',(2.46956253587978,3.25876677211529,16.6127063571564));
#36380=CARTESIAN_POINT('Ctrl Pts',(-1.40764010337363,3.8388604211456,16.8116392955199));
#36381=CARTESIAN_POINT('Ctrl Pts',(-3.99079281651019,0.889872288227052,
17.0105722338833));
#36382=CARTESIAN_POINT('Ctrl Pts',(-2.90519160811827,-2.87717947194522,
17.2095051722467));
#36383=CARTESIAN_POINT('Ctrl Pts',(0.851165411244564,-3.99922710487472,
17.4084381106102));
#36384=CARTESIAN_POINT('Ctrl Pts',(3.82504221077387,-1.44476713676006,17.6073710489736));
#36385=CARTESIAN_POINT('Ctrl Pts',(3.28254037176988,2.43787380751438,17.806303987337));
#36386=CARTESIAN_POINT('Ctrl Pts',(-0.277615706683554,4.07936631268466,
18.0052369257005));
#36387=CARTESIAN_POINT('Ctrl Pts',(-3.58255840789535,1.97067887989953,18.2041698640639));
#36388=CARTESIAN_POINT('Ctrl Pts',(-3.59403892943819,-1.94966257781868,
18.4031028024274));
#36389=CARTESIAN_POINT('Ctrl Pts',(-0.301503175830768,-4.07767039234755,
18.6020357407908));
#36390=CARTESIAN_POINT('Ctrl Pts',(3.26820581365757,-2.45705733617242,18.8009686791542));
#36391=CARTESIAN_POINT('Ctrl Pts',(3.83343838792988,1.42233966393734,18.9999016175177));
#36392=CARTESIAN_POINT('Ctrl Pts',(0.874573679959915,3.99417336528914,19.1988345558811));
#36393=CARTESIAN_POINT('Ctrl Pts',(-2.88829057535421,2.89414539130014,19.3977674942445));
#36394=CARTESIAN_POINT('Ctrl Pts',(-3.99593621570884,-0.866483556480068,
19.596700432608));
#36395=CARTESIAN_POINT('Ctrl Pts',(-1.43009958434302,-3.83055024409362,
19.7956333709714));
#36396=CARTESIAN_POINT('Ctrl Pts',(2.45043407577578,-3.27317473318194,19.9945663093349));
#36397=CARTESIAN_POINT('Ctrl Pts',(4.07827258525759,0.293245143182466,20.1934992476983));
#36398=CARTESIAN_POINT('Ctrl Pts',(1.95693662536422,3.59008343050296,20.3924321860618));
#36399=CARTESIAN_POINT('Ctrl Pts',(-1.96342004259136,3.58654175076973,20.5913651244252));
#36400=CARTESIAN_POINT('Ctrl Pts',(-4.07879576764655,0.285875986211559,
20.7902980627886));
#36401=CARTESIAN_POINT('Ctrl Pts',(-2.44451605938545,-3.27759686799192,
20.989231001152));
#36402=CARTESIAN_POINT('Ctrl Pts',(1.43701834022598,-3.82796006817182,21.1881639395155));
#36403=CARTESIAN_POINT('Ctrl Pts',(3.99749526744709,-0.85926223028944,21.3870968778789));
#36404=CARTESIAN_POINT('Ctrl Pts',(2.88305667961953,2.89935926986721,21.5860298162423));
#36405=CARTESIAN_POINT('Ctrl Pts',(-0.881788979099839,3.99258665403793,
21.7849627546059));
#36406=CARTESIAN_POINT('Ctrl Pts',(-3.83600203327774,1.41541103371171,21.9838956929692));
#36407=CARTESIAN_POINT('Ctrl Pts',(-3.26376103442727,-2.46295836420717,
22.1828286313327));
#36408=CARTESIAN_POINT('Ctrl Pts',(0.30887027395015,-4.07711897637704,22.3817615696961));
#36409=CARTESIAN_POINT('Ctrl Pts',(3.59755573975958,-1.94316563704349,22.5806945080596));
#36410=CARTESIAN_POINT('Ctrl Pts',(3.57899191075299,1.97714867838221,22.779627446423));
#36411=CARTESIAN_POINT('Ctrl Pts',(0.270244599062885,4.07986125381013,22.9785603847864));
#36412=CARTESIAN_POINT('Ctrl Pts',(-3.28693979722906,2.43193888966304,23.1774933231499));
#36413=CARTESIAN_POINT('Ctrl Pts',(-3.82242554230984,-1.45167591671186,
23.3764262615133));
#36414=CARTESIAN_POINT('Ctrl Pts',(-0.843938164034378,-4.00075847420837,
23.5753591998767));
#36415=CARTESIAN_POINT('Ctrl Pts',(2.91038539296211,-2.87192563589251,23.7742921382402));
#36416=CARTESIAN_POINT('Ctrl Pts',(3.98917846904379,0.897081454373756,23.9732250766036));
#36417=CARTESIAN_POINT('Ctrl Pts',(1.40070170053866,3.8413974982774,24.1721580149671));
#36418=CARTESIAN_POINT('Ctrl Pts',(-2.47544648891397,3.25429941372752,24.3710909533305));
#36419=CARTESIAN_POINT('Ctrl Pts',(-4.07590550298146,-0.324490869562239,
24.5700238916939));
#36420=CARTESIAN_POINT('Ctrl Pts',(-1.92936611713726,-3.60497522594906,
24.7689568300574));
#36421=CARTESIAN_POINT('Ctrl Pts',(1.9908482836132,-3.57138952024253,24.9678897684208));
#36422=CARTESIAN_POINT('Ctrl Pts',(4.08086683519371,-0.254609243900974,
25.1668227067842));
#36423=CARTESIAN_POINT('Ctrl Pts',(2.41932601167626,3.29623446418644,25.3657556451477));
#36424=CARTESIAN_POINT('Ctrl Pts',(-1.46631217817726,3.81683489160756,25.5646885835111));
#36425=CARTESIAN_POINT('Ctrl Pts',(-4.00396293765922,0.828601706198546,
25.7636215218746));
#36426=CARTESIAN_POINT('Ctrl Pts',(-2.86075242355659,-2.92136878274188,
25.962554460238));
#36427=CARTESIAN_POINT('Ctrl Pts',(0.912360757761685,-3.98571171076888,
26.1614873986014));
#36428=CARTESIAN_POINT('Ctrl Pts',(3.84673655987073,-1.38597180080177,26.3604203369649));
#36429=CARTESIAN_POINT('Ctrl Pts',(3.24479001000817,2.4878982665324,26.5593532753283));
#36430=CARTESIAN_POINT('Ctrl Pts',(-0.340106700660735,4.07463218288835,
26.7582862136918));
#36431=CARTESIAN_POINT('Ctrl Pts',(-3.61234178013069,1.91553826826458,26.9572191520552));
#36432=CARTESIAN_POINT('Ctrl Pts',(-3.56373469086466,-2.00451865713232,
27.1561520904186));
#36433=CARTESIAN_POINT('Ctrl Pts',(-0.238970150300533,-4.0818124970323,
27.355085028782));
#36434=CARTESIAN_POINT('Ctrl Pts',(3.30548073238998,-2.4066776106206,27.5540179671455));
#36435=CARTESIAN_POINT('Ctrl Pts',(3.81118819815281,1.4809269097172,27.7529509055089));
#36436=CARTESIAN_POINT('Ctrl Pts',(0.813253081967926,4.00710861074834,27.9518838438724));
#36437=CARTESIAN_POINT('Ctrl Pts',(-2.93230927793693,2.84953720666863,28.1508167822358));
#36438=CARTESIAN_POINT('Ctrl Pts',(-3.98218643011584,-0.927626664917013,
28.3497497205993));
#36439=CARTESIAN_POINT('Ctrl Pts',(-1.37122155078066,-3.85201913966408,
28.5486826589627));
#36440=CARTESIAN_POINT('Ctrl Pts',(2.50031351423257,-3.23523296289614,28.7476155973261));
#36441=CARTESIAN_POINT('Ctrl Pts',(4.07329903479392,0.355717537957839,28.9465485356896));
#36442=CARTESIAN_POINT('Ctrl Pts',(1.90168229346025,3.61965529414108,29.145481474053));
#36443=CARTESIAN_POINT('Ctrl Pts',(-2.01815959821697,3.55602753501551,29.3444144124164));
#36444=CARTESIAN_POINT('Ctrl Pts',(-4.08269822544072,0.223327547890934,
29.5433473507799));
#36445=CARTESIAN_POINT('Ctrl Pts',(-2.393993872213,-3.31467846607637,29.7422802891433));
#36446=CARTESIAN_POINT('Ctrl Pts',(1.49551989674303,-3.80548554485619,29.9412132275068));
#36447=CARTESIAN_POINT('Ctrl Pts',(4.01019544728766,-0.797892516706975,
30.1401461658702));
#36448=CARTESIAN_POINT('Ctrl Pts',(2.8382801499021,2.94320671790745,30.3390791042336));
#36449=CARTESIAN_POINT('Ctrl Pts',(-0.942878951689648,3.97860267884648,
30.5380120425971));
#36450=CARTESIAN_POINT('Ctrl Pts',(-3.85724516009308,1.35645116705405,30.7369449809605));
#36451=CARTESIAN_POINT('Ctrl Pts',(-3.22562841271805,-2.51269204972075,
30.935877919324));
#36452=CARTESIAN_POINT('Ctrl Pts',(0.371323152238799,-4.07190607827283,
31.1348108576874));
#36453=CARTESIAN_POINT('Ctrl Pts',(3.62691566059552,-1.88779839617231,31.3337437960508));
#36454=CARTESIAN_POINT('Ctrl Pts',(3.54826816585965,2.03177090657653,31.5326767344143));
#36455=CARTESIAN_POINT('Ctrl Pts',(0.207681666353341,4.08352400741375,31.7316096727777));
#36456=CARTESIAN_POINT('Ctrl Pts',(-3.32382753019483,2.38127498268946,31.9305426111411));
#36457=CARTESIAN_POINT('Ctrl Pts',(-3.79972701545007,-1.51009092498523,
32.1294755495046));
#36458=CARTESIAN_POINT('Ctrl Pts',(-0.782520235955546,-4.01322340195306,
32.328408487868));
#36459=CARTESIAN_POINT('Ctrl Pts',(2.9540609426459,-2.82698141854484,32.5273414262314));
#36460=CARTESIAN_POINT('Ctrl Pts',(3.97496050958118,0.958117394129718,32.7262743645949));
#36461=CARTESIAN_POINT('Ctrl Pts',(1.34166086649601,3.86241454442386,32.9252073029583));
#36462=CARTESIAN_POINT('Ctrl Pts',(-2.52503369124243,3.21597650049785,33.1241402413218));
#36463=CARTESIAN_POINT('Ctrl Pts',(-4.07045333377795,-0.38692331436581,
33.3230731796852));
#36464=CARTESIAN_POINT('Ctrl Pts',(-1.87388678025847,-3.63412277288981,
33.5220061180486));
#36465=CARTESIAN_POINT('Ctrl Pts',(2.04535238235562,-3.54045669732818,33.720939056412));
#36466=CARTESIAN_POINT('Ctrl Pts',(4.08428983082642,-0.192032735416775,
33.9198719947756));
#36467=CARTESIAN_POINT('Ctrl Pts',(2.36852112880191,3.3329277904093,34.1188049331389));
#36468=CARTESIAN_POINT('Ctrl Pts',(-1.5246397804968,3.79391269448716,34.3177378715024));
#36469=CARTESIAN_POINT('Ctrl Pts',(-4.01619243028494,0.767136465425386,
34.5166708098658));
#36470=CARTESIAN_POINT('Ctrl Pts',(-2.81564117849665,-2.96487179277909,
34.7156037482293));
#36471=CARTESIAN_POINT('Ctrl Pts',(0.973341768490662,-3.97125997579838,
34.9145366865927));
#36472=CARTESIAN_POINT('Ctrl Pts',(3.8675272167539,-1.32685086627251,35.1134696249562));
#36473=CARTESIAN_POINT('Ctrl Pts',(3.20627736795542,2.53733825758359,35.3124025633196));
#36474=CARTESIAN_POINT('Ctrl Pts',(-0.402517795281907,4.06894082264232,
35.511335501683));
#36475=CARTESIAN_POINT('Ctrl Pts',(-3.64127652519993,1.85994764997906,35.7102684400464));
#36476=CARTESIAN_POINT('Ctrl Pts',(-3.53259324412043,-2.0589038261282,35.9092013784099));
#36477=CARTESIAN_POINT('Ctrl Pts',(-0.176380984849015,-4.08499568445078,
36.1081343167733));
#36478=CARTESIAN_POINT('Ctrl Pts',(3.34197911308852,-2.35573249778373,36.3070672551368));
#36479=CARTESIAN_POINT('Ctrl Pts',(3.78804266736189,1.53916624959495,36.5060001935002));
#36480=CARTESIAN_POINT('Ctrl Pts',(0.751741430954012,4.0191024888065,36.7049331318636));
#36481=CARTESIAN_POINT('Ctrl Pts',(-2.97563910948809,2.80425959604127,36.9038660702271));
#36482=CARTESIAN_POINT('Ctrl Pts',(-3.96750113199172,-0.988551850799671,
37.1027990085905));
#36483=CARTESIAN_POINT('Ctrl Pts',(-1.31202138353558,-3.87258310284293,
37.301731946954));
#36484=CARTESIAN_POINT('Ctrl Pts',(2.54960556749285,-3.19653115591342,37.5006648853174));
#36485=CARTESIAN_POINT('Ctrl Pts',(4.06736856819161,0.418106362963447,37.6995978236809));
#36486=CARTESIAN_POINT('Ctrl Pts',(1.84598120786055,3.64837681833342,37.8985307620442));
#36487=CARTESIAN_POINT('Ctrl Pts',(-2.07242503480969,3.52467791048579,38.0974637004078));
#36488=CARTESIAN_POINT('Ctrl Pts',(-4.0856415657996,0.160726665959935,38.2963966387711));
#36489=CARTESIAN_POINT('Ctrl Pts',(-2.34290926230782,-3.3509814065453,38.4953295771346));
#36490=CARTESIAN_POINT('Ctrl Pts',(1.5536700900277,-3.78211694123996,38.694262515498));
#36491=CARTESIAN_POINT('Ctrl Pts',(4.02195359031618,-0.736335510109945,
38.8931954538615));
#36492=CARTESIAN_POINT('Ctrl Pts',(2.79283673182646,2.98636302520864,39.0921283922249));
#36493=CARTESIAN_POINT('Ctrl Pts',(-1.00374721358184,3.96368347627922,39.2910613305884));
#36494=CARTESIAN_POINT('Ctrl Pts',(-3.87758251988644,1.29717370417073,39.4899942689517));
#36495=CARTESIAN_POINT('Ctrl Pts',(-3.18673725693753,-2.56183748892951,
39.6889272073153));
#36496=CARTESIAN_POINT('Ctrl Pts',(0.433687349425391,-4.06573266647945,
39.8878601456786));
#36497=CARTESIAN_POINT('Ctrl Pts',(3.65542630739156,-1.83199518874432,40.0867930840421));
#36498=CARTESIAN_POINT('Ctrl Pts',(3.51670552180105,2.08593024760723,40.2857260224055));
#36499=CARTESIAN_POINT('Ctrl Pts',(0.145080153377126,4.08619978216286,40.484658960769));
#36500=CARTESIAN_POINT('Ctrl Pts',(-3.35995399040756,2.33010469112103,40.6835918991324));
#36501=CARTESIAN_POINT('Ctrl Pts',(-3.77609830574217,-1.56825286709605,
40.8825248374958));
#36502=CARTESIAN_POINT('Ctrl Pts',(-0.720990444685169,-4.02455053491554,
41.0814577758593));
#36503=CARTESIAN_POINT('Ctrl Pts',(2.99718051531959,-2.78174701105068,41.2803907142227));
#36504=CARTESIAN_POINT('Ctrl Pts',(3.9595440561214,1.01964576599861,41.4793236525862));
#36505=CARTESIAN_POINT('Ctrl Pts',(1.28281295705702,3.88114366634645,41.6782565909495));
#36506=CARTESIAN_POINT('Ctrl Pts',(-2.57500755361336,3.17958857837247,41.8771895293131));
#36507=CARTESIAN_POINT('Ctrl Pts',(-4.0621147000577,-0.454817851921865,
42.0761224676764));
#36508=CARTESIAN_POINT('Ctrl Pts',(-2.56886110523792,-2.5838694518668,42.2087444265854));
#36509=CARTESIAN_POINT('Ctrl Pts',(-1.53687260224456,-3.09613266190232,
42.2750554060399));
#36510=CARTESIAN_POINT('Ctrl Pts',(-1.86645400133787,2.62012303844274,7.00322156819806));
#36511=CARTESIAN_POINT('Ctrl Pts',(-2.74041061257865,1.997626899089,7.0695770455426));
#36512=CARTESIAN_POINT('Ctrl Pts',(-3.80025934494349,-0.179501204411249,
7.20224350234162));
#36513=CARTESIAN_POINT('Ctrl Pts',(-1.89809237229961,-3.30104156426044,
7.40122093859512));
#36514=CARTESIAN_POINT('Ctrl Pts',(1.75033879183918,-3.37766291872948,7.60015387695855));
#36515=CARTESIAN_POINT('Ctrl Pts',(3.78874883692714,-0.353950369213094,
7.79908681532199));
#36516=CARTESIAN_POINT('Ctrl Pts',(2.34462897392162,2.99761246260044,7.99801975368543));
#36517=CARTESIAN_POINT('Ctrl Pts',(-1.25517146953415,3.59217513842517,8.19695269204886));
#36518=CARTESIAN_POINT('Ctrl Pts',(-3.70095537602795,0.885102952948687,
8.39588563041231));
#36519=CARTESIAN_POINT('Ctrl Pts',(-2.74450292932235,-2.63599675282763,
8.59481856877575));
#36520=CARTESIAN_POINT('Ctrl Pts',(0.735019325049069,-3.73363101754262,
8.79375150713918));
#36521=CARTESIAN_POINT('Ctrl Pts',(3.53881629779805,-1.39901612008267,8.99268444550262));
#36522=CARTESIAN_POINT('Ctrl Pts',(3.08937315587434,2.22177005300786,9.19161738386606));
#36523=CARTESIAN_POINT('Ctrl Pts',(-0.200149810864368,3.80004717549578,
9.3905503222295));
#36524=CARTESIAN_POINT('Ctrl Pts',(-3.30567149883918,1.88493714980744,9.58948326059294));
#36525=CARTESIAN_POINT('Ctrl Pts',(-3.37227577980602,-1.76301114979847,
9.78841619895636));
#36526=CARTESIAN_POINT('Ctrl Pts',(-0.338730933097911,-3.79021165389004,
9.98734913731983));
#36527=CARTESIAN_POINT('Ctrl Pts',(3.00621041944956,-2.33305531494441,10.1862820756832));
#36528=CARTESIAN_POINT('Ctrl Pts',(3.58752910607548,1.26889034228732,10.3852150140467));
#36529=CARTESIAN_POINT('Ctrl Pts',(0.870815925397089,3.70433883892876,10.5841479524101));
#36530=CARTESIAN_POINT('Ctrl Pts',(-2.64644222848811,2.73437212425091,10.7830808907735));
#36531=CARTESIAN_POINT('Ctrl Pts',(-3.73081407650405,-0.749315416829459,
10.9820138291369));
#36532=CARTESIAN_POINT('Ctrl Pts',(-1.38543162233216,-3.54415382593228,
11.1809467675004));
#36533=CARTESIAN_POINT('Ctrl Pts',(2.23358439312533,-3.08083559997405,11.3798797058638));
#36534=CARTESIAN_POINT('Ctrl Pts',(3.79925615786297,0.214708774655039,11.5788126442273));
#36535=CARTESIAN_POINT('Ctrl Pts',(1.87225451730644,3.31287038929909,11.7777455825907));
#36536=CARTESIAN_POINT('Ctrl Pts',(-1.77591918454253,3.36549524737367,11.9766785209541));
#36537=CARTESIAN_POINT('Ctrl Pts',(-3.79148233256386,0.32420507008613,12.1756114593176));
#36538=CARTESIAN_POINT('Ctrl Pts',(-2.32151858988368,-3.01512829587034,
12.374544397681));
#36539=CARTESIAN_POINT('Ctrl Pts',(1.28262771288672,-3.58264055637097,12.5734773360444));
#36540=CARTESIAN_POINT('Ctrl Pts',(3.70764854672028,-0.85661511733405,12.7724102744079));
#36541=CARTESIAN_POINT('Ctrl Pts',(2.72421126934337,2.65690048083118,12.9713432127713));
#36542=CARTESIAN_POINT('Ctrl Pts',(-0.763605773387818,3.72791542664558,
13.1702761511348));
#36543=CARTESIAN_POINT('Ctrl Pts',(-3.54943656817764,1.37184082667385,13.3692090894982));
#36544=CARTESIAN_POINT('Ctrl Pts',(-3.0722542406453,-2.24537326208117,13.5681420278616));
#36545=CARTESIAN_POINT('Ctrl Pts',(0.229265333024543,-3.79840553553036,
13.7670749662251));
#36546=CARTESIAN_POINT('Ctrl Pts',(3.32002024707132,-1.85954638670049,13.9660079045885));
#36547=CARTESIAN_POINT('Ctrl Pts',(3.35866550245346,1.78880218243472,14.164940842952));
#36548=CARTESIAN_POINT('Ctrl Pts',(0.309674340768458,3.79269679883976,14.3638737813154));
#36549=CARTESIAN_POINT('Ctrl Pts',(-3.02400184575466,2.30994806048298,14.5628067196789));
#36550=CARTESIAN_POINT('Ctrl Pts',(-3.57769943142826,-1.29634639800277,
14.7617396580423));
#36551=CARTESIAN_POINT('Ctrl Pts',(-0.842401716518874,-3.71090373807563,
14.9606725964057));
#36552=CARTESIAN_POINT('Ctrl Pts',(2.66731971394778,-2.71401045481454,15.1596055347691));
#36553=CARTESIAN_POINT('Ctrl Pts',(3.72496204373251,0.777884938798361,15.3585384731326));
#36554=CARTESIAN_POINT('Ctrl Pts',(1.35822988608424,3.55466718298702,15.557471411496));
#36555=CARTESIAN_POINT('Ctrl Pts',(-2.25712916101158,3.06362777696122,15.7564043498595));
#36556=CARTESIAN_POINT('Ctrl Pts',(-3.7974991416244,-0.243818528047306,
15.9553372882229));
#36557=CARTESIAN_POINT('Ctrl Pts',(-1.84681095199157,-3.32712135529518,
16.1542702265864));
#36558=CARTESIAN_POINT('Ctrl Pts',(1.80165891510899,-3.35178644290854,16.3532031649498));
#36559=CARTESIAN_POINT('Ctrl Pts',(3.79385557686611,-0.295139064068223,
16.5521361033133));
#36560=CARTESIAN_POINT('Ctrl Pts',(2.29834361397166,3.03283099386907,16.7510690416766));
#36561=CARTESIAN_POINT('Ctrl Pts',(-1.31004604878593,3.57270577508387,16.9500019800401));
#36562=CARTESIAN_POINT('Ctrl Pts',(-3.71410444208186,0.828175946623051,
17.1489349184035));
#36563=CARTESIAN_POINT('Ctrl Pts',(-2.70376979034626,-2.677699782662,17.347867856767));
#36564=CARTESIAN_POINT('Ctrl Pts',(0.792152682487336,-3.7219539670562,17.5468007951304));
#36565=CARTESIAN_POINT('Ctrl Pts',(3.55984560446539,-1.3445990025378,17.7457337334939));
#36566=CARTESIAN_POINT('Ctrl Pts',(3.05495632989659,2.26885191841203,17.9446666718573));
#36567=CARTESIAN_POINT('Ctrl Pts',(-0.25836814307153,3.79653698887591,18.1435996102207));
#36568=CARTESIAN_POINT('Ctrl Pts',(-3.33417361125188,1.83404840047608,18.3425325485842));
#36569=CARTESIAN_POINT('Ctrl Pts',(-3.34485816893761,-1.8144891939465,18.5414654869476));
#36570=CARTESIAN_POINT('Ctrl Pts',(-0.280599453828384,-3.79495864954658,
18.740398425311));
#36571=CARTESIAN_POINT('Ctrl Pts',(3.04161561079433,-2.28670542078106,18.9393313636745));
#36572=CARTESIAN_POINT('Ctrl Pts',(3.56765966054535,1.32372646410603,19.1382643020379));
#36573=CARTESIAN_POINT('Ctrl Pts',(0.813938016583792,3.71725061173132,19.3371972404014));
#36574=CARTESIAN_POINT('Ctrl Pts',(-2.68804053459405,2.69348942630865,19.5361301787648));
#36575=CARTESIAN_POINT('Ctrl Pts',(-3.71889124076811,-0.8064087949641,19.7350631171283));
#36576=CARTESIAN_POINT('Ctrl Pts',(-1.33094837618574,-3.56497175657617,
19.9339960554916));
#36577=CARTESIAN_POINT('Ctrl Pts',(2.28054136216125,-3.04624002677545,20.1329289938551));
#36578=CARTESIAN_POINT('Ctrl Pts',(3.79551909140992,0.272913964465135,20.3318619322185));
#36579=CARTESIAN_POINT('Ctrl Pts',(1.8212589195482,3.34117691139266,20.530794870582));
#36580=CARTESIAN_POINT('Ctrl Pts',(-1.8272928305604,3.33788078226886,20.7297278089454));
#36581=CARTESIAN_POINT('Ctrl Pts',(-3.79600600068437,0.266055723534535,
20.9286607473089));
#36582=CARTESIAN_POINT('Ctrl Pts',(-2.27503365179541,-3.05035556754547,
21.1275936856723));
#36583=CARTESIAN_POINT('Ctrl Pts',(1.33738744309295,-3.56256116190508,21.3265266240357));
#36584=CARTESIAN_POINT('Ctrl Pts',(3.72034220082859,-0.799688135457281,
21.5254595623992));
#36585=CARTESIAN_POINT('Ctrl Pts',(2.6831695136488,2.69834181791016,21.7243925007626));
#36586=CARTESIAN_POINT('Ctrl Pts',(-0.820653066905469,3.7157739098384,21.923325439126));
#36587=CARTESIAN_POINT('Ctrl Pts',(-3.57004556405178,1.31727820746093,22.1222583774895));
#36588=CARTESIAN_POINT('Ctrl Pts',(-3.03747899557971,-2.29219732062257,
22.3211913158529));
#36589=CARTESIAN_POINT('Ctrl Pts',(0.287455778651096,-3.79444546417224,
22.5201242542163));
#36590=CARTESIAN_POINT('Ctrl Pts',(3.34813115288769,-1.80844269699657,22.7190571925798));
#36591=CARTESIAN_POINT('Ctrl Pts',(3.33085438535164,1.84006963695426,22.9179901309432));
#36592=CARTESIAN_POINT('Ctrl Pts',(0.251508086732996,3.79699761490117,23.1169230693067));
#36593=CARTESIAN_POINT('Ctrl Pts',(-3.0590507357933,2.26332847839188,23.3158560076701));
#36594=CARTESIAN_POINT('Ctrl Pts',(-3.55741035402456,-1.35102878516191,
23.5147889460336));
#36595=CARTESIAN_POINT('Ctrl Pts',(-0.785426512475196,-3.72337916397971,
23.7137218843969));
#36596=CARTESIAN_POINT('Ctrl Pts',(2.70860348135616,-2.67281020389449,23.9126548227604));
#36597=CARTESIAN_POINT('Ctrl Pts',(3.71260202003901,0.83488528916224,24.1115877611238));
#36598=CARTESIAN_POINT('Ctrl Pts',(1.30358869708293,3.57506695239331,24.3105206994873));
#36599=CARTESIAN_POINT('Ctrl Pts',(-2.3038196226511,3.02867336494793,24.5094536378507));
#36600=CARTESIAN_POINT('Ctrl Pts',(-3.79331612292701,-0.301993372111428,
24.7083865762142));
#36601=CARTESIAN_POINT('Ctrl Pts',(-1.7955999210022,-3.35503623362761,24.9073195145776));
#36602=CARTESIAN_POINT('Ctrl Pts',(1.85281942552575,-3.32377908135478,25.1062524529411));
#36603=CARTESIAN_POINT('Ctrl Pts',(3.79793347763706,-0.23695675702724,25.3051853913045));
#36604=CARTESIAN_POINT('Ctrl Pts',(2.25159007243797,3.06770098786632,25.5041183296679));
#36605=CARTESIAN_POINT('Ctrl Pts',(-1.36465029001659,3.55220731253327,25.7030512680313));
#36606=CARTESIAN_POINT('Ctrl Pts',(-3.72636145659287,0.771153357041461,
25.9019842063948));
#36607=CARTESIAN_POINT('Ctrl Pts',(-2.66241164915182,-2.7188253742596,26.1009171447582));
#36608=CARTESIAN_POINT('Ctrl Pts',(0.849105252762015,-3.70937561794287,
26.2998500831217));
#36609=CARTESIAN_POINT('Ctrl Pts',(3.58003584787151,-1.28988004605551,26.4987830214851));
#36610=CARTESIAN_POINT('Ctrl Pts',(3.01982326417359,2.31540809759601,26.6977159598485));
#36611=CARTESIAN_POINT('Ctrl Pts',(-0.316526531389901,3.79213108425639,
26.896648898212));
#36612=CARTESIAN_POINT('Ctrl Pts',(-3.36189205222476,1.78273078013626,27.0955818365754));
#36613=CARTESIAN_POINT('Ctrl Pts',(-3.31665497416533,-1.86554200906911,
27.294514774939));
#36614=CARTESIAN_POINT('Ctrl Pts',(-0.222401948075185,-3.79881357515075,
27.4934477133024));
#36615=CARTESIAN_POINT('Ctrl Pts',(3.07630619675248,-2.23981860628926,27.6923806516658));
#36616=CARTESIAN_POINT('Ctrl Pts',(3.54695211382774,1.37825175765173,27.8913135900291));
#36617=CARTESIAN_POINT('Ctrl Pts',(0.756868878729541,3.72928903487889,28.0902465283926));
#36618=CARTESIAN_POINT('Ctrl Pts',(-2.72900734653197,2.65197400210329,28.2891794667561));
#36619=CARTESIAN_POINT('Ctrl Pts',(-3.70609475092345,-0.863312748912513,
28.4881124051195));
#36620=CARTESIAN_POINT('Ctrl Pts',(-1.27615245566332,-3.58495217752786,
28.6870453434829));
#36621=CARTESIAN_POINT('Ctrl Pts',(2.32696257530329,-3.01092882320308,28.8859782818464));
#36622=CARTESIAN_POINT('Ctrl Pts',(3.79089036556033,0.331055043095624,29.0849112202098));
#36623=CARTESIAN_POINT('Ctrl Pts',(1.7698354633568,3.36869850801491,29.2838441585732));
#36624=CARTESIAN_POINT('Ctrl Pts',(-1.87823720077816,3.3094821683868,29.4827770969367));
#36625=CARTESIAN_POINT('Ctrl Pts',(-3.79963789451971,0.207843873585611,
29.6817100353001));
#36626=CARTESIAN_POINT('Ctrl Pts',(-2.22801425278663,-3.08486623610115,
29.8806429736635));
#36627=CARTESIAN_POINT('Ctrl Pts',(1.39183298835648,-3.54164483507025,30.079575912027));
#36628=CARTESIAN_POINT('Ctrl Pts',(3.73216185585201,-0.742573287279,30.2785088503904));
#36629=CARTESIAN_POINT('Ctrl Pts',(2.64149741600532,2.73914924867091,30.4774417887539));
#36630=CARTESIAN_POINT('Ctrl Pts',(-0.877507569004345,3.70275946715383,
30.6763747271173));
#36631=CARTESIAN_POINT('Ctrl Pts',(-3.58981586917566,1.26240612746925,30.8753076654808));
#36632=CARTESIAN_POINT('Ctrl Pts',(-3.00199017263393,-2.33848288611794,
31.0742406038442));
#36633=CARTESIAN_POINT('Ctrl Pts',(0.345578693905692,-3.78959398505641,
31.2731735422076));
#36634=CARTESIAN_POINT('Ctrl Pts',(3.37545550105851,-1.75691416000643,31.4721064805712));
#36635=CARTESIAN_POINT('Ctrl Pts',(3.3022607693379,1.89090481424875,31.6710394189345));
#36636=CARTESIAN_POINT('Ctrl Pts',(0.193282747315501,3.80040642364043,31.8699723572979));
#36637=CARTESIAN_POINT('Ctrl Pts',(-3.09338098022485,2.216177185254,32.0689052956615));
#36638=CARTESIAN_POINT('Ctrl Pts',(-3.53628555418785,-1.40539378271698,
32.2678382340249));
#36639=CARTESIAN_POINT('Ctrl Pts',(-0.728266792592632,-3.73497987733052,
32.4667711723883));
#36640=CARTESIAN_POINT('Ctrl Pts',(2.74925093176247,-2.63098204468606,32.6657041107517));
#36641=CARTESIAN_POINT('Ctrl Pts',(3.69936981560612,0.891689504614469,32.8646370491151));
#36642=CARTESIAN_POINT('Ctrl Pts',(1.24864126331116,3.59462685140112,33.0635699874787));
#36643=CARTESIAN_POINT('Ctrl Pts',(-2.34996886088683,2.99300744371268,33.262502925842));
#36644=CARTESIAN_POINT('Ctrl Pts',(-3.78824196177939,-0.360097270568816,
33.4614358642054));
#36645=CARTESIAN_POINT('Ctrl Pts',(-1.74396705980911,-3.38216293214238,
33.660368802569));
#36646=CARTESIAN_POINT('Ctrl Pts',(1.90354466348184,-3.29499088305067,33.8593017409324));
#36647=CARTESIAN_POINT('Ctrl Pts',(3.80111915122855,-0.17871878306637,34.0582346792959));
#36648=CARTESIAN_POINT('Ctrl Pts',(2.20430757749551,3.10185030410124,34.2571676176593));
#36649=CARTESIAN_POINT('Ctrl Pts',(-1.41893394161954,3.5308743498711,34.4561005560226));
#36650=CARTESIAN_POINT('Ctrl Pts',(-3.73774305793726,0.713949604733199,
34.6550334943861));
#36651=CARTESIAN_POINT('Ctrl Pts',(-2.62042804254318,-2.75931224748304,
34.8539664327496));
#36652=CARTESIAN_POINT('Ctrl Pts',(0.90585834750904,-3.69592584605102,35.052899371113));
#36653=CARTESIAN_POINT('Ctrl Pts',(3.59938505356419,-1.23485806529853,35.2518323094765));
#36654=CARTESIAN_POINT('Ctrl Pts',(2.98398076833351,2.36142033095977,35.4507652478398));
#36655=CARTESIAN_POINT('Ctrl Pts',(-0.374610559908926,3.7868343155833,35.6496981862033));
#36656=CARTESIAN_POINT('Ctrl Pts',(-3.3888207027795,1.73099435286343,35.8486311245668));
#36657=CARTESIAN_POINT('Ctrl Pts',(-3.28767261627215,-1.91615656287791,
36.0475640629301));
#36658=CARTESIAN_POINT('Ctrl Pts',(-0.164152194675816,-3.80177606683461,
36.2464970012937));
#36659=CARTESIAN_POINT('Ctrl Pts',(3.11027408336399,-2.1924056037633,36.445429939657));
#36660=CARTESIAN_POINT('Ctrl Pts',(3.52541130159383,1.43245326619635,36.6443628780206));
#36661=CARTESIAN_POINT('Ctrl Pts',(0.699621933880535,3.74045135720976,36.843295816384));
#36662=CARTESIAN_POINT('Ctrl Pts',(-2.76933304802493,2.60983556433168,37.0422287547475));
#36663=CARTESIAN_POINT('Ctrl Pts',(-3.69242760920404,-0.920013889243654,
37.2411616931107));
#36664=CARTESIAN_POINT('Ctrl Pts',(-1.22105673552787,-3.60409040657181,
37.4400946314743));
#36665=CARTESIAN_POINT('Ctrl Pts',(2.37283712765188,-2.9749102775556,37.6390275698377));
#36666=CARTESIAN_POINT('Ctrl Pts',(3.7853710681766,0.389118345988962,37.8379605082012));
#36667=CARTESIAN_POINT('Ctrl Pts',(1.71799622765437,3.39542872065456,38.0368934465646));
#36668=CARTESIAN_POINT('Ctrl Pts',(-1.92874032343257,3.28030606602396,38.235826384928));
#36669=CARTESIAN_POINT('Ctrl Pts',(-3.80237716814379,0.149583216029986,
38.4347593232914));
#36670=CARTESIAN_POINT('Ctrl Pts',(-2.1804714247586,-3.1186522326827,38.633692261655));
#36671=CARTESIAN_POINT('Ctrl Pts',(1.44595153099118,-3.51989641602498,38.8326252000182));
#36672=CARTESIAN_POINT('Ctrl Pts',(3.74310478705912,-0.685284131425703,
39.0315581383817));
#36673=CARTESIAN_POINT('Ctrl Pts',(2.59920466649454,2.77931345664184,39.2304910767451));
#36674=CARTESIAN_POINT('Ctrl Pts',(-0.934155731980976,3.68887463797949,
39.4294240151087));
#36675=CARTESIAN_POINT('Ctrl Pts',(-3.60874320562774,1.20723847073212,39.628356953472));
#36676=CARTESIAN_POINT('Ctrl Pts',(-2.9657954060591,-2.38422098941366,39.8272898918356));
#36677=CARTESIAN_POINT('Ctrl Pts',(0.403619076468115,-3.78384858628005,
40.0262228301989));
#36678=CARTESIAN_POINT('Ctrl Pts',(3.40198945678621,-1.70497988275374,40.2251557685625));
#36679=CARTESIAN_POINT('Ctrl Pts',(3.27288641644818,1.9413091971248,40.4240887069258));
#36680=CARTESIAN_POINT('Ctrl Pts',(0.135021502466078,3.80289668242824,40.6230216452892));
#36681=CARTESIAN_POINT('Ctrl Pts',(-3.12700273222302,2.16855461601647,40.8219545836528));
#36682=CARTESIAN_POINT('Ctrl Pts',(-3.51429506264349,-1.45952325961196,
41.020887522016));
#36683=CARTESIAN_POINT('Ctrl Pts',(-0.671002965181634,-3.74552168112398,
41.2198204603797));
#36684=CARTESIAN_POINT('Ctrl Pts',(2.78938095197937,-2.58888381470178,41.418753398743));
#36685=CARTESIAN_POINT('Ctrl Pts',(3.68502221077952,0.948952011033468,41.6176863371064));
#36686=CARTESIAN_POINT('Ctrl Pts',(1.19387337835599,3.61205745181745,41.8166192754698));
#36687=CARTESIAN_POINT('Ctrl Pts',(-2.39647795137431,2.95914235739577,42.0155522138333));
#36688=CARTESIAN_POINT('Ctrl Pts',(-3.78048145955207,-0.423284565706465,
42.2144851521968));
#36689=CARTESIAN_POINT('Ctrl Pts',(-2.39075764659687,-2.40472543932513,
42.3471071111058));
#36690=CARTESIAN_POINT('Ctrl Pts',(-1.43031864127241,-2.88147257990253,
42.4134180905602));
#36691=CARTESIAN_POINT('Ctrl Pts',(-0.0207003078980803,-3.22266463217033,
35.));
#36692=CARTESIAN_POINT('Ctrl Pts',(0.390179082935768,-3.27339145921622,
35.));
#36693=CARTESIAN_POINT('Ctrl Pts',(0.778605604939595,-3.24434960842915,
35.));
#36694=CARTESIAN_POINT('Ctrl Pts',(1.56185674874276,-3.03916248926379,35.));
#36695=CARTESIAN_POINT('Ctrl Pts',(1.94872076465658,-2.8510360063766,35.));
#36696=CARTESIAN_POINT('Ctrl Pts',(2.68187385484571,-2.32275572829235,35.));
#36697=CARTESIAN_POINT('Ctrl Pts',(3.01817343547782,-1.96309141773522,35.));
#36698=CARTESIAN_POINT('Ctrl Pts',(3.49494789802835,-1.17980918440496,35.));
#36699=CARTESIAN_POINT('Ctrl Pts',(3.65560097307578,-0.759652858975631,
35.));
#36700=CARTESIAN_POINT('Ctrl Pts',(3.78646125695233,0.0823884449927741,
35.));
#36701=CARTESIAN_POINT('Ctrl Pts',(3.79123516462661,0.443182121773422,35.));
#36702=CARTESIAN_POINT('Ctrl Pts',(3.70863692495699,1.13742209958287,35.));
#36703=CARTESIAN_POINT('Ctrl Pts',(3.62486017046094,1.47282751573001,35.));
#36704=CARTESIAN_POINT('Ctrl Pts',(3.49931608640154,1.79133081339196,35.));
#36705=CARTESIAN_POINT('Ctrl Pts',(-3.8864130136037,0.610157723633211,38.));
#36706=CARTESIAN_POINT('Ctrl Pts',(-3.772631518137,1.05264935984635,38.));
#36707=CARTESIAN_POINT('Ctrl Pts',(-3.57839040445375,1.47494376323108,38.));
#36708=CARTESIAN_POINT('Ctrl Pts',(-3.03687080404268,2.26623247828738,38.));
#36709=CARTESIAN_POINT('Ctrl Pts',(-2.67423971095682,2.62879046566468,38.));
#36710=CARTESIAN_POINT('Ctrl Pts',(-1.89042756718785,3.13666861491962,38.));
#36711=CARTESIAN_POINT('Ctrl Pts',(-1.4826961685891,3.30719881404164,38.));
#36712=CARTESIAN_POINT('Ctrl Pts',(-0.560741755968393,3.47676848286895,
38.));
#36713=CARTESIAN_POINT('Ctrl Pts',(-0.0952693922769644,3.47380165091183,
38.));
#36714=CARTESIAN_POINT('Ctrl Pts',(0.654416143995199,3.32412025485652,38.));
#36715=CARTESIAN_POINT('Ctrl Pts',(0.949919393676216,3.22355758047029,38.));
#36716=CARTESIAN_POINT('Ctrl Pts',(1.41353731808283,2.98479081726645,38.));
#36717=CARTESIAN_POINT('Ctrl Pts',(1.66686279531448,2.83000589683937,38.));
#36718=CARTESIAN_POINT('Ctrl Pts',(1.92910760072171,2.58159390771144,38.));
#36719=CARTESIAN_POINT('Origin',(-9.5,-25.9558441227157,44.142135623731));
#36720=CARTESIAN_POINT('',(-9.5,-25.9558441227157,49.142135623731));
#36721=CARTESIAN_POINT('',(-10.,-25.9558441227157,49.642135623731));
#36722=CARTESIAN_POINT('Origin',(-9.5,-25.9558441227157,49.642135623731));
#36723=CARTESIAN_POINT('',(-10.,-22.0667568261897,48.031222920257));
#36724=CARTESIAN_POINT('Origin',(-10.,-25.9558441227157,44.142135623731));
#36725=CARTESIAN_POINT('',(-9.5,-22.420310216783,47.6776695296637));
#36726=CARTESIAN_POINT('Origin',(-9.5,-22.0667568261897,48.031222920257));
#36727=CARTESIAN_POINT('Origin',(-9.5,-25.9558441227157,44.142135623731));
#36728=CARTESIAN_POINT('Origin',(-9.5,-27.9350288425444,53.8994949366117));
#36729=CARTESIAN_POINT('',(-10.,-10.8535533905933,36.8180194846605));
#36730=CARTESIAN_POINT('',(-9.5,-11.2071067811866,36.4644660940673));
#36731=CARTESIAN_POINT('Origin',(-9.5,-10.8535533905933,36.8180194846605));
#36732=CARTESIAN_POINT('',(-9.5,-28.2885822331377,53.5459415460184));
#36733=CARTESIAN_POINT('',(-10.,-27.9350288425444,53.8994949366117));
#36734=CARTESIAN_POINT('Origin',(-9.5,-7.67157287525382,40.));
#36735=CARTESIAN_POINT('',(-10.,-7.67157287525382,35.5));
#36736=CARTESIAN_POINT('',(-9.5,-7.67157287525382,35.));
#36737=CARTESIAN_POINT('Origin',(-9.5,-7.67157287525382,35.5));
#36738=CARTESIAN_POINT('Origin',(-9.5,-7.67157287525382,40.));
#36739=CARTESIAN_POINT('Origin',(-10.,-7.67157287525382,40.));
#36740=CARTESIAN_POINT('Origin',(-9.5,-28.4068542494924,35.5));
#36741=CARTESIAN_POINT('',(-10.,0.499999999999998,35.5));
#36742=CARTESIAN_POINT('',(-9.5,0.499999999999998,35.));
#36743=CARTESIAN_POINT('Origin',(-9.5,0.499999999999998,35.5));
#36744=CARTESIAN_POINT('',(-9.5,-28.4068542494924,35.));
#36745=CARTESIAN_POINT('',(-10.,-28.4068542494924,35.5));
#36746=CARTESIAN_POINT('Origin',(-2.,0.499999999999998,35.5));
#36747=CARTESIAN_POINT('',(-2.,8.5,35.5));
#36748=CARTESIAN_POINT('',(-2.,8.,35.));
#36749=CARTESIAN_POINT('Origin',(-2.,8.,35.5));
#36750=CARTESIAN_POINT('Origin',(-2.,0.499999999999998,35.));
#36751=CARTESIAN_POINT('Origin',(-2.,0.499999999999998,35.5));
#36752=CARTESIAN_POINT('Origin',(0.,8.,35.5));
#36753=CARTESIAN_POINT('',(2.,8.5,35.5));
#36754=CARTESIAN_POINT('',(2.,8.,35.));
#36755=CARTESIAN_POINT('Origin',(2.,8.,35.5));
#36756=CARTESIAN_POINT('',(0.,8.,35.));
#36757=CARTESIAN_POINT('',(0.,8.5,35.5));
#36758=CARTESIAN_POINT('Origin',(2.,0.499999999999998,35.5));
#36759=CARTESIAN_POINT('',(10.,0.499999999999998,35.5));
#36760=CARTESIAN_POINT('',(9.5,0.499999999999998,35.));
#36761=CARTESIAN_POINT('Origin',(9.5,0.499999999999998,35.5));
#36762=CARTESIAN_POINT('Origin',(2.,0.499999999999998,35.));
#36763=CARTESIAN_POINT('Origin',(2.,0.499999999999998,35.5));
#36764=CARTESIAN_POINT('Origin',(9.5,-28.4068542494924,35.5));
#36765=CARTESIAN_POINT('',(10.,-7.67157287525382,35.5));
#36766=CARTESIAN_POINT('',(9.5,-7.67157287525382,35.));
#36767=CARTESIAN_POINT('Origin',(9.5,-7.67157287525382,35.5));
#36768=CARTESIAN_POINT('',(9.5,-28.4068542494924,35.));
#36769=CARTESIAN_POINT('',(10.,-28.4068542494924,35.5));
#36770=CARTESIAN_POINT('Origin',(9.5,-7.67157287525382,40.));
#36771=CARTESIAN_POINT('',(10.,-10.8535533905933,36.8180194846605));
#36772=CARTESIAN_POINT('',(9.5,-11.2071067811866,36.4644660940673));
#36773=CARTESIAN_POINT('Origin',(9.5,-10.8535533905933,36.8180194846605));
#36774=CARTESIAN_POINT('Origin',(9.5,-7.67157287525382,40.));
#36775=CARTESIAN_POINT('Origin',(10.,-7.67157287525382,40.));
#36776=CARTESIAN_POINT('Origin',(9.5,-27.9350288425444,53.8994949366117));
#36777=CARTESIAN_POINT('',(10.,-22.0667568261897,48.031222920257));
#36778=CARTESIAN_POINT('',(9.5,-22.420310216783,47.6776695296637));
#36779=CARTESIAN_POINT('Origin',(9.5,-22.0667568261897,48.031222920257));
#36780=CARTESIAN_POINT('',(9.5,-28.2885822331377,53.5459415460184));
#36781=CARTESIAN_POINT('',(10.,-27.9350288425444,53.8994949366117));
#36782=CARTESIAN_POINT('Origin',(9.5,-25.9558441227157,44.142135623731));
#36783=CARTESIAN_POINT('',(10.,-25.9558441227157,49.642135623731));
#36784=CARTESIAN_POINT('',(9.5,-25.9558441227157,49.142135623731));
#36785=CARTESIAN_POINT('Origin',(9.5,-25.9558441227157,49.642135623731));
#36786=CARTESIAN_POINT('Origin',(9.5,-25.9558441227157,44.142135623731));
#36787=CARTESIAN_POINT('Origin',(10.,-25.9558441227157,44.142135623731));
#36788=CARTESIAN_POINT('Origin',(9.5,-74.8566017177982,49.642135623731));
#36789=CARTESIAN_POINT('',(10.,-92.6421356237309,49.642135623731));
#36790=CARTESIAN_POINT('',(9.5,-92.6421356237309,49.142135623731));
#36791=CARTESIAN_POINT('Origin',(9.5,-92.6421356237309,49.642135623731));
#36792=CARTESIAN_POINT('',(9.5,-74.8566017177982,49.142135623731));
#36793=CARTESIAN_POINT('',(10.,-74.8566017177982,49.642135623731));
#36794=CARTESIAN_POINT('Origin',(0.,-92.6421356237309,49.642135623731));
#36795=CARTESIAN_POINT('',(-10.,-92.6421356237309,49.642135623731));
#36796=CARTESIAN_POINT('',(-9.5,-92.6421356237309,49.142135623731));
#36797=CARTESIAN_POINT('Origin',(-9.5,-92.6421356237309,49.642135623731));
#36798=CARTESIAN_POINT('Origin',(0.,-92.6421356237309,49.142135623731));
#36799=CARTESIAN_POINT('Origin',(0.,-92.6421356237309,49.642135623731));
#36800=CARTESIAN_POINT('Origin',(-9.5,-74.8566017177982,49.642135623731));
#36801=CARTESIAN_POINT('',(-10.,-74.8566017177982,49.642135623731));
#36802=CARTESIAN_POINT('',(-9.5,-74.8566017177982,49.142135623731));
#36803=CARTESIAN_POINT('Origin',(2.,0.499999999999998,39.2855339059327));
#36804=CARTESIAN_POINT('',(2.,8.5,37.5));
#36805=CARTESIAN_POINT('',(2.,8.5,39.2855339059327));
#36806=CARTESIAN_POINT('',(10.,0.499999999999998,37.5));
#36807=CARTESIAN_POINT('Origin',(2.,0.499999999999998,37.5));
#36808=CARTESIAN_POINT('',(10.,0.499999999999998,39.2855339059327));
#36809=CARTESIAN_POINT('Origin',(0.,8.5,35.));
#36810=CARTESIAN_POINT('',(-2.,8.5,37.5));
#36811=CARTESIAN_POINT('',(-2.,8.5,39.2855339059327));
#36812=CARTESIAN_POINT('',(0.,8.5,37.5));
#36813=CARTESIAN_POINT('Origin',(-2.,0.499999999999998,39.2855339059327));
#36814=CARTESIAN_POINT('',(-10.,0.499999999999998,37.5));
#36815=CARTESIAN_POINT('',(-10.,0.499999999999998,39.2855339059327));
#36816=CARTESIAN_POINT('Origin',(-2.,0.499999999999998,37.5));
#36817=CARTESIAN_POINT('Origin',(-10.,-47.0710678118655,43.5710678118655));
#36818=CARTESIAN_POINT('',(-10.,-92.6421356237309,51.642135623731));
#36819=CARTESIAN_POINT('',(-10.,-92.6421356237309,47.8566017177982));
#36820=CARTESIAN_POINT('',(-10.,-24.7132034355964,51.642135623731));
#36821=CARTESIAN_POINT('',(-10.,-34.8566017177982,51.642135623731));
#36822=CARTESIAN_POINT('',(-10.,-21.531222920257,50.3241161390704));
#36823=CARTESIAN_POINT('Origin',(-10.,-24.7132034355964,47.142135623731));
#36824=CARTESIAN_POINT('',(-10.,-10.3180194846605,39.110912703474));
#36825=CARTESIAN_POINT('',(-10.,-19.889087296526,48.6819805153395));
#36826=CARTESIAN_POINT('',(-10.,-6.42893218813451,37.5));
#36827=CARTESIAN_POINT('Origin',(-10.,-6.42893218813451,43.));
#36828=CARTESIAN_POINT('',(-10.,-19.2855339059327,37.5));
#36829=CARTESIAN_POINT('Origin',(0.,-102.642135623731,49.142135623731));
#36830=CARTESIAN_POINT('',(0.,-25.9558441227157,49.142135623731));
#36831=CARTESIAN_POINT('Origin',(0.,-7.67157287525382,40.));
#36832=CARTESIAN_POINT('',(0.,-11.2071067811866,36.4644660940673));
#36833=CARTESIAN_POINT('',(0.,-7.67157287525382,35.));
#36834=CARTESIAN_POINT('Origin',(0.,-23.8847763108502,49.142135623731));
#36835=CARTESIAN_POINT('',(0.,-22.420310216783,47.6776695296637));
#36836=CARTESIAN_POINT('Origin',(0.,-25.9558441227157,44.142135623731));
#36837=CARTESIAN_POINT('Origin',(9.5,-24.7132034355964,47.142135623731));
#36838=CARTESIAN_POINT('',(9.5,-24.7132034355964,52.142135623731));
#36839=CARTESIAN_POINT('',(10.,-24.7132034355964,51.642135623731));
#36840=CARTESIAN_POINT('Origin',(9.5,-24.7132034355964,51.642135623731));
#36841=CARTESIAN_POINT('',(10.,-21.531222920257,50.3241161390704));
#36842=CARTESIAN_POINT('Origin',(10.,-24.7132034355964,47.142135623731));
#36843=CARTESIAN_POINT('',(9.5,-21.1776695296637,50.6776695296637));
#36844=CARTESIAN_POINT('Origin',(9.5,-21.531222920257,50.3241161390704));
#36845=CARTESIAN_POINT('Origin',(9.5,-24.7132034355964,47.142135623731));
#36846=CARTESIAN_POINT('Origin',(9.5,-19.889087296526,48.6819805153395));
#36847=CARTESIAN_POINT('',(10.,-10.3180194846605,39.110912703474));
#36848=CARTESIAN_POINT('',(9.5,-9.96446609406726,39.4644660940673));
#36849=CARTESIAN_POINT('Origin',(9.5,-10.3180194846605,39.110912703474));
#36850=CARTESIAN_POINT('',(9.5,-19.5355339059327,49.0355339059327));
#36851=CARTESIAN_POINT('',(10.,-19.889087296526,48.6819805153395));
#36852=CARTESIAN_POINT('Origin',(9.5,-6.42893218813451,43.));
#36853=CARTESIAN_POINT('',(10.,-6.42893218813451,37.5));
#36854=CARTESIAN_POINT('',(9.5,-6.42893218813451,38.));
#36855=CARTESIAN_POINT('Origin',(9.5,-6.42893218813451,37.5));
#36856=CARTESIAN_POINT('Origin',(9.5,-6.42893218813451,43.));
#36857=CARTESIAN_POINT('Origin',(10.,-6.42893218813451,43.));
#36858=CARTESIAN_POINT('Origin',(9.5,-19.2855339059327,37.5));
#36859=CARTESIAN_POINT('',(9.5,0.499999999999998,38.));
#36860=CARTESIAN_POINT('Origin',(9.5,0.499999999999998,37.5));
#36861=CARTESIAN_POINT('',(9.5,-19.2855339059327,38.));
#36862=CARTESIAN_POINT('',(10.,-19.2855339059327,37.5));
#36863=CARTESIAN_POINT('Origin',(2.,0.499999999999998,37.5));
#36864=CARTESIAN_POINT('',(2.,8.,38.));
#36865=CARTESIAN_POINT('Origin',(2.,8.,37.5));
#36866=CARTESIAN_POINT('Origin',(2.,0.499999999999998,38.));
#36867=CARTESIAN_POINT('Origin',(0.,8.,37.5));
#36868=CARTESIAN_POINT('',(-2.,8.,38.));
#36869=CARTESIAN_POINT('Origin',(-2.,8.,37.5));
#36870=CARTESIAN_POINT('',(0.,8.,38.));
#36871=CARTESIAN_POINT('Origin',(-2.,0.499999999999998,37.5));
#36872=CARTESIAN_POINT('',(-9.5,0.499999999999998,38.));
#36873=CARTESIAN_POINT('Origin',(-9.5,0.499999999999998,37.5));
#36874=CARTESIAN_POINT('Origin',(-2.,0.499999999999998,38.));
#36875=CARTESIAN_POINT('Origin',(-9.5,-19.2855339059327,37.5));
#36876=CARTESIAN_POINT('',(-9.5,-6.42893218813451,38.));
#36877=CARTESIAN_POINT('Origin',(-9.5,-6.42893218813451,37.5));
#36878=CARTESIAN_POINT('',(-9.5,-19.2855339059327,38.));
#36879=CARTESIAN_POINT('Origin',(-9.5,-6.42893218813451,43.));
#36880=CARTESIAN_POINT('',(-9.5,-9.96446609406726,39.4644660940673));
#36881=CARTESIAN_POINT('Origin',(-9.5,-10.3180194846605,39.110912703474));
#36882=CARTESIAN_POINT('Origin',(-9.5,-6.42893218813451,43.));
#36883=CARTESIAN_POINT('Origin',(-9.5,-19.889087296526,48.6819805153395));
#36884=CARTESIAN_POINT('',(-9.5,-21.1776695296637,50.6776695296637));
#36885=CARTESIAN_POINT('Origin',(-9.5,-21.531222920257,50.3241161390704));
#36886=CARTESIAN_POINT('',(-9.5,-19.5355339059327,49.0355339059327));
#36887=CARTESIAN_POINT('Origin',(-9.5,-24.7132034355964,47.142135623731));
#36888=CARTESIAN_POINT('',(-9.5,-24.7132034355964,52.142135623731));
#36889=CARTESIAN_POINT('Origin',(-9.5,-24.7132034355964,51.642135623731));
#36890=CARTESIAN_POINT('Origin',(-9.5,-24.7132034355964,47.142135623731));
#36891=CARTESIAN_POINT('Origin',(-9.5,-34.8566017177982,51.642135623731));
#36892=CARTESIAN_POINT('',(-9.5,-92.6421356237309,52.142135623731));
#36893=CARTESIAN_POINT('Origin',(-9.5,-92.6421356237309,51.642135623731));
#36894=CARTESIAN_POINT('',(-9.5,-34.8566017177982,52.142135623731));
#36895=CARTESIAN_POINT('Origin',(0.,-92.6421356237309,51.642135623731));
#36896=CARTESIAN_POINT('',(10.,-92.6421356237309,51.642135623731));
#36897=CARTESIAN_POINT('',(9.5,-92.6421356237309,52.142135623731));
#36898=CARTESIAN_POINT('Origin',(9.5,-92.6421356237309,51.642135623731));
#36899=CARTESIAN_POINT('Origin',(0.,-92.6421356237309,52.142135623731));
#36900=CARTESIAN_POINT('Origin',(0.,-92.6421356237309,51.642135623731));
#36901=CARTESIAN_POINT('Origin',(9.5,-34.8566017177982,51.642135623731));
#36902=CARTESIAN_POINT('',(10.,-34.8566017177982,51.642135623731));
#36903=CARTESIAN_POINT('',(9.5,-34.8566017177982,52.142135623731));
#36904=CARTESIAN_POINT('Origin',(0.,-22.6421356237309,52.142135623731));
#36905=CARTESIAN_POINT('',(0.,-24.7132034355964,52.142135623731));
#36906=CARTESIAN_POINT('Origin',(0.,-6.42893218813451,43.));
#36907=CARTESIAN_POINT('',(0.,-9.96446609406726,39.4644660940673));
#36908=CARTESIAN_POINT('',(0.,-6.42893218813451,38.));
#36909=CARTESIAN_POINT('Origin',(0.,-8.5,38.));
#36910=CARTESIAN_POINT('',(0.,-21.1776695296637,50.6776695296637));
#36911=CARTESIAN_POINT('Origin',(0.,-24.7132034355964,47.142135623731));
#36912=CARTESIAN_POINT('Origin',(10.,-47.0710678118655,43.5710678118655));
#36913=CARTESIAN_POINT('',(10.,-92.6421356237309,47.8566017177982));
#36914=CARTESIAN_POINT('Origin',(0.,-92.6421356237309,47.8566017177982));
#36915=CARTESIAN_POINT('Origin',(0.,-9.74264068711929,35.));
#36916=CARTESIAN_POINT('Origin',(0.,8.5,38.));
#42654=UNCERTAINTY_MEASURE_WITH_UNIT(LENGTH_MEASURE(0.01),#42668,
'DISTANCE_ACCURACY_VALUE',
'Maximum model space distance between geometric entities at asserted c
onnectivities');
#42656=UNCERTAINTY_MEASURE_WITH_UNIT(LENGTH_MEASURE(0.01),#42668,
'DISTANCE_ACCURACY_VALUE',
'Maximum model space distance between geometric entities at asserted c
onnectivities');
#42665=(
GEOMETRIC_REPRESENTATION_CONTEXT(3)
GLOBAL_UNCERTAINTY_ASSIGNED_CONTEXT((#42654))
GLOBAL_UNIT_ASSIGNED_CONTEXT((#42668,#42670,#42671))
REPRESENTATION_CONTEXT('','3D')
);
#42667=(
GEOMETRIC_REPRESENTATION_CONTEXT(3)
GLOBAL_UNCERTAINTY_ASSIGNED_CONTEXT((#42656))
GLOBAL_UNIT_ASSIGNED_CONTEXT((#42668,#42670,#42671))
REPRESENTATION_CONTEXT('','3D')
);
#42668=(
LENGTH_UNIT()
NAMED_UNIT(*)
SI_UNIT(.MILLI.,.METRE.)
);
#42670=(
NAMED_UNIT(*)
PLANE_ANGLE_UNIT()
SI_UNIT($,.RADIAN.)
);
#42671=(
NAMED_UNIT(*)
SI_UNIT($,.STERADIAN.)
SOLID_ANGLE_UNIT()
);
#42680=SHAPE_DEFINITION_REPRESENTATION(#42690,#42709);
#42690=PRODUCT_DEFINITION_SHAPE('',$,#42720);
#42709=SHAPE_REPRESENTATION('',(#4317),#42665);
#42711=PRODUCT_DEFINITION_CONTEXT('part definition',#42743,'design');
#42720=PRODUCT_DEFINITION('Handle','Handle',#42730,#42711);
#42730=PRODUCT_DEFINITION_FORMATION('',$,#42753);
#42743=APPLICATION_CONTEXT(
'Core Data for Automotive Mechanical Design Process');
#42744=PRODUCT_CONTEXT('part definition',#42743,'mechanical');
#42753=PRODUCT('Handle','Handle',$,(#42744));
#42756=PRESENTATION_STYLE_ASSIGNMENT((#42758));
#42758=SURFACE_STYLE_USAGE(.BOTH.,#42760);
#42760=SURFACE_SIDE_STYLE('',(#42762));
#42762=SURFACE_STYLE_FILL_AREA(#42764);
#42764=FILL_AREA_STYLE('Opaque(160,160,160)',(#42766));
#42766=FILL_AREA_STYLE_COLOUR('Opaque(160,160,160)',#42768);
#42768=COLOUR_RGB('Opaque(160,160,160)', 0.09019608, 0.27058824, 0.51372549);
ENDSEC;
END-ISO-10303-21;
